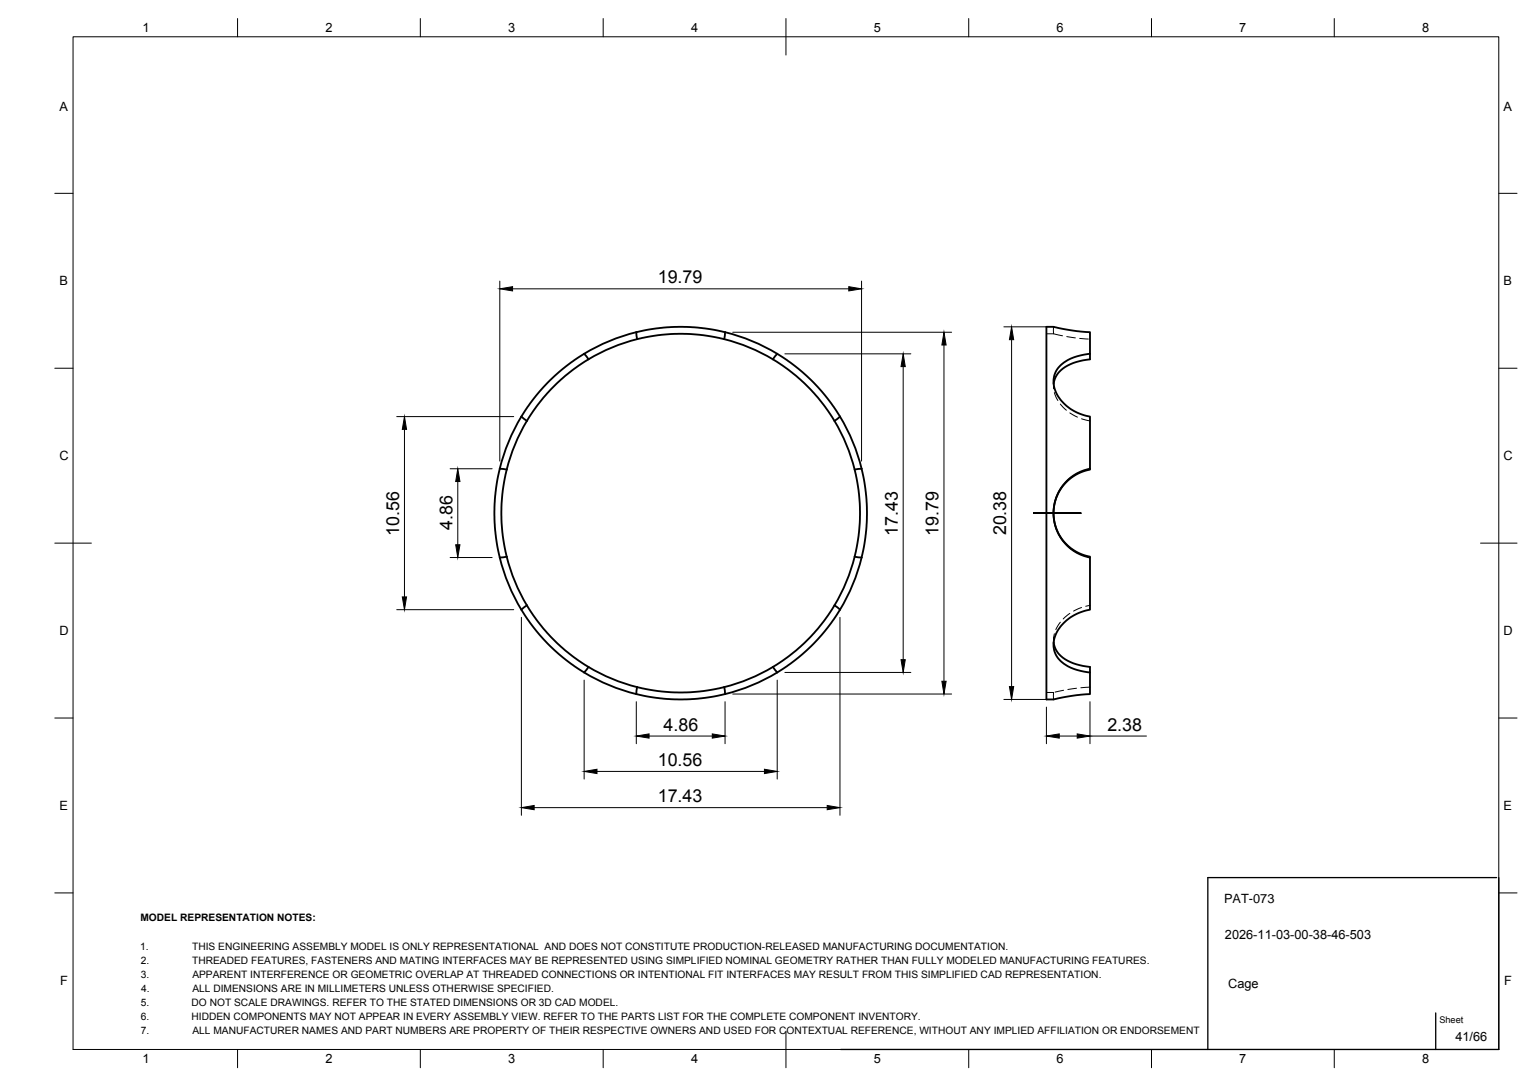
ISO-10303-21;
HEADER;
/* Generated by software containing ST-Developer
 * from STEP Tools, Inc. (www.steptools.com) 
 */

FILE_DESCRIPTION(
/* description */ ('Manual piston pump'),
/* implementation_level */ '2;1');

FILE_NAME(
/* name */ 'Cage.step',
/* time_stamp */ '2026-11-02T16:54:23-08:00',
/* author */ (''),
/* organization */ (''),
/* preprocessor_version */ 'ST-DEVELOPER v20.2',
/* originating_system */ 'Autodesk Translation Framework v15.17.0.0',
/* authorisation */ '');

FILE_SCHEMA (('AUTOMOTIVE_DESIGN { 1 0 10303 214 3 1 1 }'));
ENDSEC;

DATA;
#10=MECHANICAL_DESIGN_GEOMETRIC_PRESENTATION_REPRESENTATION('',(#721),#19043);
#500=SPHERICAL_SURFACE('',#10763,0.247676);
#501=SPHERICAL_SURFACE('',#10779,0.247676);
#502=SPHERICAL_SURFACE('',#10784,0.247676);
#503=SPHERICAL_SURFACE('',#10789,0.247676);
#504=SPHERICAL_SURFACE('',#10794,0.247676);
#505=SPHERICAL_SURFACE('',#10799,0.247676);
#506=SPHERICAL_SURFACE('',#10804,0.247676);
#507=SPHERICAL_SURFACE('',#10812,0.247676);
#588=SHAPE_REPRESENTATION_RELATIONSHIP('SRR','None',#19335,#651);
#651=ADVANCED_BREP_SHAPE_REPRESENTATION('',(#791),#19002);
#721=STYLED_ITEM('',(#19661),#791);
#791=MANIFOLD_SOLID_BREP('Continuous crown cage',#9507);
#950=FACE_BOUND('',#2270,.T.);
#1051=B_SPLINE_CURVE_WITH_KNOTS('',3,(#15858,#15859,#15860,#15861,#15862,
#15863,#15864,#15865,#15866,#15867,#15868,#15869,#15870,#15871,#15872,#15873,
#15874,#15875,#15876,#15877,#15878,#15879),.UNSPECIFIED.,.F.,.F.,(4,2,2,
2,2,2,2,2,2,2,4),(0.0473477652366656,0.126350602536658,0.189525903804987,
0.252701205073317,0.313298422430275,0.373895639787233,0.434492857144191,
0.495090074501149,0.558265375769478,0.621440677037807,0.7004435143378),
 .UNSPECIFIED.);
#1052=B_SPLINE_CURVE_WITH_KNOTS('',3,(#15883,#15884,#15885,#15886,#15887,
#15888,#15889,#15890,#15891,#15892,#15893,#15894,#15895,#15896,#15897,#15898,
#15899,#15900,#15901,#15902,#15903,#15904),.UNSPECIFIED.,.F.,.F.,(4,2,2,
2,2,2,2,2,2,2,4),(0.0464897534940957,0.0852567806515119,0.170513561303024,
0.246687263103517,0.308657850341199,0.370628437578881,0.432599024816563,
0.494569612054245,0.570743313854739,0.656000094506251,0.694767121663666),
 .UNSPECIFIED.);
#1053=B_SPLINE_CURVE_WITH_KNOTS('',3,(#15910,#15911,#15912,#15913,#15914,
#15915,#15916,#15917,#15918,#15919,#15920,#15921,#15922,#15923,#15924,#15925,
#15926,#15927,#15928,#15929,#15930,#15931),.UNSPECIFIED.,.F.,.F.,(4,2,2,
2,2,2,2,2,2,2,4),(0.0464897534940957,0.0852567806515118,0.170513561303024,
0.246687263103517,0.308657850341199,0.370628437578881,0.432599024816563,
0.494569612054245,0.570743313854738,0.65600009450625,0.694767121663666),
 .UNSPECIFIED.);
#1054=B_SPLINE_CURVE_WITH_KNOTS('',3,(#15935,#15936,#15937,#15938,#15939,
#15940,#15941,#15942,#15943,#15944,#15945,#15946,#15947,#15948,#15949,#15950,
#15951,#15952,#15953,#15954,#15955,#15956),.UNSPECIFIED.,.F.,.F.,(4,2,2,
2,2,2,2,2,2,2,4),(0.0464897534940957,0.0852567806515119,0.170513561303024,
0.246687263103517,0.308657850341199,0.370628437578881,0.432599024816563,
0.494569612054245,0.570743313854739,0.656000094506251,0.694767121663666),
 .UNSPECIFIED.);
#1055=B_SPLINE_CURVE_WITH_KNOTS('',3,(#15960,#15961,#15962,#15963,#15964,
#15965,#15966,#15967,#15968,#15969,#15970,#15971),.UNSPECIFIED.,.F.,.F.,
(4,2,2,2,2,4),(0.0464897534940957,0.0852567806515119,0.170513561303024,
0.246687263103517,0.308657850341199,0.370628437578881),.UNSPECIFIED.);
#1056=B_SPLINE_CURVE_WITH_KNOTS('',3,(#15976,#15977,#15978,#15979,#15980,
#15981,#15982,#15983,#15984,#15985,#15986,#15987),.UNSPECIFIED.,.F.,.F.,
(4,2,2,2,2,4),(0.370628437578881,0.432599024816563,0.494569612054245,0.570743313854738,
0.65600009450625,0.694767121663666),.UNSPECIFIED.);
#1057=B_SPLINE_CURVE_WITH_KNOTS('',3,(#15991,#15992,#15993,#15994,#15995,
#15996,#15997,#15998,#15999,#16000,#16001,#16002,#16003,#16004,#16005,#16006,
#16007,#16008,#16009,#16010,#16011,#16012),.UNSPECIFIED.,.F.,.F.,(4,2,2,
2,2,2,2,2,2,2,4),(0.0464897534940957,0.0852567806515121,0.170513561303024,
0.246687263103518,0.308657850341199,0.370628437578881,0.432599024816563,
0.494569612054245,0.570743313854738,0.65600009450625,0.694767121663666),
 .UNSPECIFIED.);
#1058=B_SPLINE_CURVE_WITH_KNOTS('',3,(#16016,#16017,#16018,#16019,#16020,
#16021,#16022,#16023,#16024,#16025,#16026,#16027,#16028,#16029,#16030,#16031,
#16032,#16033,#16034,#16035,#16036,#16037),.UNSPECIFIED.,.F.,.F.,(4,2,2,
2,2,2,2,2,2,2,4),(0.0464897534940957,0.0852567806515119,0.170513561303024,
0.246687263103517,0.308657850341199,0.370628437578881,0.432599024816563,
0.494569612054245,0.570743313854738,0.65600009450625,0.694767121663667),
 .UNSPECIFIED.);
#1059=B_SPLINE_CURVE_WITH_KNOTS('',3,(#16041,#16042,#16043,#16044,#16045,
#16046,#16047,#16048,#16049,#16050,#16051,#16052,#16053,#16054,#16055,#16056,
#16057,#16058,#16059,#16060,#16061,#16062),.UNSPECIFIED.,.F.,.F.,(4,2,2,
2,2,2,2,2,2,2,4),(0.0464897534940957,0.0852567806515119,0.170513561303024,
0.246687263103517,0.308657850341199,0.370628437578881,0.432599024816563,
0.494569612054245,0.570743313854738,0.65600009450625,0.694767121663666),
 .UNSPECIFIED.);
#1060=B_SPLINE_CURVE_WITH_KNOTS('',3,(#16066,#16067,#16068,#16069,#16070,
#16071,#16072,#16073,#16074,#16075,#16076,#16077,#16078,#16079,#16080,#16081,
#16082,#16083,#16084,#16085,#16086,#16087),.UNSPECIFIED.,.F.,.F.,(4,2,2,
2,2,2,2,2,2,2,4),(0.0464897534940957,0.0852567806515119,0.170513561303024,
0.246687263103517,0.308657850341199,0.370628437578881,0.432599024816563,
0.494569612054245,0.570743313854739,0.656000094506251,0.694767121663667),
 .UNSPECIFIED.);
#1061=B_SPLINE_CURVE_WITH_KNOTS('',3,(#16095,#16096,#16097,#16098,#16099,
#16100,#16101,#16102,#16103,#16104,#16105,#16106,#16107,#16108,#16109,#16110,
#16111,#16112,#16113,#16114,#16115,#16116),.UNSPECIFIED.,.F.,.F.,(4,2,2,
2,2,2,2,2,2,2,4),(0.0473477652366656,0.126350602536658,0.189525903804987,
0.252701205073316,0.313298422430274,0.373895639787232,0.434492857144191,
0.495090074501149,0.558265375769478,0.621440677037807,0.7004435143378),
 .UNSPECIFIED.);
#1062=B_SPLINE_CURVE_WITH_KNOTS('',3,(#16124,#16125,#16126,#16127,#16128,
#16129,#16130,#16131,#16132,#16133,#16134,#16135,#16136,#16137,#16138,#16139,
#16140,#16141,#16142,#16143,#16144,#16145),.UNSPECIFIED.,.F.,.F.,(4,2,2,
2,2,2,2,2,2,2,4),(0.0473477652366656,0.126350602536658,0.189525903804987,
0.252701205073317,0.313298422430275,0.373895639787233,0.434492857144191,
0.495090074501149,0.558265375769478,0.621440677037807,0.7004435143378),
 .UNSPECIFIED.);
#1063=B_SPLINE_CURVE_WITH_KNOTS('',3,(#16154,#16155,#16156,#16157,#16158,
#16159,#16160,#16161,#16162,#16163,#16164,#16165),.UNSPECIFIED.,.F.,.F.,
(4,2,2,2,2,4),(0.0473477652366656,0.126350602536658,0.189525903804987,0.252701205073316,
0.313298422430275,0.373895639787233),.UNSPECIFIED.);
#1064=B_SPLINE_CURVE_WITH_KNOTS('',3,(#16167,#16168,#16169,#16170,#16171,
#16172,#16173,#16174,#16175,#16176,#16177,#16178),.UNSPECIFIED.,.F.,.F.,
(4,2,2,2,2,4),(0.373895639787233,0.434492857144191,0.495090074501149,0.558265375769478,
0.621440677037807,0.7004435143378),.UNSPECIFIED.);
#1065=B_SPLINE_CURVE_WITH_KNOTS('',3,(#16185,#16186,#16187,#16188,#16189,
#16190,#16191,#16192,#16193,#16194,#16195,#16196,#16197,#16198,#16199,#16200,
#16201,#16202,#16203,#16204,#16205,#16206),.UNSPECIFIED.,.F.,.F.,(4,2,2,
2,2,2,2,2,2,2,4),(0.0473477652366656,0.126350602536658,0.189525903804987,
0.252701205073316,0.313298422430275,0.373895639787233,0.434492857144191,
0.495090074501149,0.558265375769478,0.621440677037807,0.7004435143378),
 .UNSPECIFIED.);
#1066=B_SPLINE_CURVE_WITH_KNOTS('',3,(#16214,#16215,#16216,#16217,#16218,
#16219,#16220,#16221,#16222,#16223,#16224,#16225,#16226,#16227,#16228,#16229,
#16230,#16231,#16232,#16233,#16234,#16235),.UNSPECIFIED.,.F.,.F.,(4,2,2,
2,2,2,2,2,2,2,4),(0.0473477652366656,0.126350602536658,0.189525903804987,
0.252701205073317,0.313298422430275,0.373895639787233,0.434492857144191,
0.495090074501149,0.558265375769478,0.621440677037807,0.7004435143378),
 .UNSPECIFIED.);
#1067=B_SPLINE_CURVE_WITH_KNOTS('',3,(#16243,#16244,#16245,#16246,#16247,
#16248,#16249,#16250,#16251,#16252,#16253,#16254,#16255,#16256,#16257,#16258,
#16259,#16260,#16261,#16262,#16263,#16264),.UNSPECIFIED.,.F.,.F.,(4,2,2,
2,2,2,2,2,2,2,4),(0.0473477652366656,0.126350602536658,0.189525903804987,
0.252701205073316,0.313298422430275,0.373895639787233,0.434492857144191,
0.495090074501149,0.558265375769478,0.621440677037807,0.7004435143378),
 .UNSPECIFIED.);
#1068=B_SPLINE_CURVE_WITH_KNOTS('',3,(#16273,#16274,#16275,#16276,#16277,
#16278,#16279,#16280,#16281,#16282,#16283,#16284,#16285,#16286,#16287,#16288,
#16289,#16290,#16291,#16292,#16293,#16294),.UNSPECIFIED.,.F.,.F.,(4,2,2,
2,2,2,2,2,2,2,4),(0.0473477652366656,0.126350602536658,0.189525903804987,
0.252701205073317,0.313298422430275,0.373895639787233,0.434492857144191,
0.495090074501149,0.558265375769478,0.621440677037807,0.7004435143378),
 .UNSPECIFIED.);
#1189=CYLINDRICAL_SURFACE('',#10766,1.019052);
#1190=CYLINDRICAL_SURFACE('',#10806,0.980948);
#1554=FACE_OUTER_BOUND('',#2252,.T.);
#1555=FACE_OUTER_BOUND('',#2253,.T.);
#1556=FACE_OUTER_BOUND('',#2254,.T.);
#1557=FACE_OUTER_BOUND('',#2255,.T.);
#1558=FACE_OUTER_BOUND('',#2256,.T.);
#1559=FACE_OUTER_BOUND('',#2257,.T.);
#1560=FACE_OUTER_BOUND('',#2258,.T.);
#1561=FACE_OUTER_BOUND('',#2259,.T.);
#1562=FACE_OUTER_BOUND('',#2260,.T.);
#1563=FACE_OUTER_BOUND('',#2261,.T.);
#1564=FACE_OUTER_BOUND('',#2262,.T.);
#1565=FACE_OUTER_BOUND('',#2263,.T.);
#1566=FACE_OUTER_BOUND('',#2264,.T.);
#1567=FACE_OUTER_BOUND('',#2265,.T.);
#1568=FACE_OUTER_BOUND('',#2266,.T.);
#1569=FACE_OUTER_BOUND('',#2267,.T.);
#1570=FACE_OUTER_BOUND('',#2268,.T.);
#1571=FACE_OUTER_BOUND('',#2269,.T.);
#1572=FACE_OUTER_BOUND('',#2271,.T.);
#2252=EDGE_LOOP('',(#7329,#7330,#7331,#7332));
#2253=EDGE_LOOP('',(#7333,#7334,#7335,#7336,#7337,#7338,#7339,#7340,#7341,
#7342,#7343,#7344,#7345,#7346,#7347,#7348,#7349,#7350,#7351,#7352));
#2254=EDGE_LOOP('',(#7353,#7354,#7355,#7356));
#2255=EDGE_LOOP('',(#7357,#7358,#7359,#7360));
#2256=EDGE_LOOP('',(#7361,#7362,#7363,#7364));
#2257=EDGE_LOOP('',(#7365,#7366,#7367,#7368));
#2258=EDGE_LOOP('',(#7369,#7370,#7371,#7372));
#2259=EDGE_LOOP('',(#7373,#7374,#7375,#7376,#7377,#7378));
#2260=EDGE_LOOP('',(#7379,#7380,#7381,#7382));
#2261=EDGE_LOOP('',(#7383,#7384,#7385,#7386));
#2262=EDGE_LOOP('',(#7387,#7388,#7389,#7390));
#2263=EDGE_LOOP('',(#7391,#7392,#7393,#7394));
#2264=EDGE_LOOP('',(#7395,#7396,#7397,#7398));
#2265=EDGE_LOOP('',(#7399,#7400,#7401,#7402));
#2266=EDGE_LOOP('',(#7403,#7404,#7405,#7406,#7407,#7408,#7409,#7410,#7411,
#7412,#7413,#7414,#7415,#7416,#7417,#7418,#7419,#7420,#7421,#7422));
#2267=EDGE_LOOP('',(#7423,#7424,#7425,#7426));
#2268=EDGE_LOOP('',(#7427,#7428,#7429,#7430));
#2269=EDGE_LOOP('',(#7431));
#2270=EDGE_LOOP('',(#7432));
#2271=EDGE_LOOP('',(#7433,#7434,#7435,#7436));
#2891=CIRCLE('',#10764,0.243053047864041);
#2892=CIRCLE('',#10765,0.243053047864041);
#2893=CIRCLE('',#10767,1.019052);
#2894=CIRCLE('',#10768,1.019052);
#2895=CIRCLE('',#10769,1.019052);
#2896=CIRCLE('',#10770,1.019052);
#2897=CIRCLE('',#10771,1.019052);
#2898=CIRCLE('',#10772,1.019052);
#2899=CIRCLE('',#10773,1.019052);
#2900=CIRCLE('',#10774,1.019052);
#2901=CIRCLE('',#10775,1.019052);
#2902=CIRCLE('',#10777,0.980948);
#2903=CIRCLE('',#10778,0.243053047864041);
#2904=CIRCLE('',#10780,0.243053047864041);
#2905=CIRCLE('',#10782,0.980948);
#2906=CIRCLE('',#10783,0.243053047864041);
#2907=CIRCLE('',#10785,0.243053047864041);
#2908=CIRCLE('',#10787,0.980948);
#2909=CIRCLE('',#10788,0.243053047864041);
#2910=CIRCLE('',#10790,0.243053047864041);
#2911=CIRCLE('',#10792,0.980948);
#2912=CIRCLE('',#10793,0.243053047864041);
#2913=CIRCLE('',#10795,0.243053047864041);
#2914=CIRCLE('',#10797,0.980948);
#2915=CIRCLE('',#10798,0.243053047864041);
#2916=CIRCLE('',#10800,0.243053047864041);
#2917=CIRCLE('',#10802,0.980948);
#2918=CIRCLE('',#10803,0.243053047864041);
#2919=CIRCLE('',#10805,0.243053047864041);
#2920=CIRCLE('',#10807,0.980948);
#2921=CIRCLE('',#10808,0.980948);
#2922=CIRCLE('',#10809,0.980948);
#2923=CIRCLE('',#10811,0.243053047864041);
#2924=CIRCLE('',#10813,0.243053047864041);
#3432=LINE('',#15973,#4036);
#3433=LINE('',#16269,#4037);
#4036=VECTOR('',#12834,1.019052);
#4037=VECTOR('',#12911,0.980948);
#4712=VERTEX_POINT('',#15856);
#4713=VERTEX_POINT('',#15857);
#4714=VERTEX_POINT('',#15880);
#4715=VERTEX_POINT('',#15882);
#4716=VERTEX_POINT('',#15907);
#4717=VERTEX_POINT('',#15909);
#4718=VERTEX_POINT('',#15932);
#4719=VERTEX_POINT('',#15934);
#4720=VERTEX_POINT('',#15957);
#4721=VERTEX_POINT('',#15959);
#4722=VERTEX_POINT('',#15972);
#4723=VERTEX_POINT('',#15975);
#4724=VERTEX_POINT('',#15988);
#4725=VERTEX_POINT('',#15990);
#4726=VERTEX_POINT('',#16013);
#4727=VERTEX_POINT('',#16015);
#4728=VERTEX_POINT('',#16038);
#4729=VERTEX_POINT('',#16040);
#4730=VERTEX_POINT('',#16063);
#4731=VERTEX_POINT('',#16065);
#4732=VERTEX_POINT('',#16090);
#4733=VERTEX_POINT('',#16094);
#4734=VERTEX_POINT('',#16119);
#4735=VERTEX_POINT('',#16123);
#4736=VERTEX_POINT('',#16148);
#4737=VERTEX_POINT('',#16152);
#4738=VERTEX_POINT('',#16153);
#4739=VERTEX_POINT('',#16180);
#4740=VERTEX_POINT('',#16184);
#4741=VERTEX_POINT('',#16209);
#4742=VERTEX_POINT('',#16213);
#4743=VERTEX_POINT('',#16238);
#4744=VERTEX_POINT('',#16242);
#4745=VERTEX_POINT('',#16267);
#4746=VERTEX_POINT('',#16270);
#4747=VERTEX_POINT('',#16272);
#5651=EDGE_CURVE('',#4712,#4713,#1051,.T.);
#5652=EDGE_CURVE('',#4714,#4712,#2891,.T.);
#5653=EDGE_CURVE('',#4715,#4714,#1052,.T.);
#5654=EDGE_CURVE('',#4713,#4715,#2892,.T.);
#5655=EDGE_CURVE('',#4716,#4714,#2893,.T.);
#5656=EDGE_CURVE('',#4716,#4717,#1053,.T.);
#5657=EDGE_CURVE('',#4718,#4717,#2894,.T.);
#5658=EDGE_CURVE('',#4718,#4719,#1054,.T.);
#5659=EDGE_CURVE('',#4720,#4719,#2895,.T.);
#5660=EDGE_CURVE('',#4720,#4721,#1055,.T.);
#5661=EDGE_CURVE('',#4721,#4722,#3432,.T.);
#5662=EDGE_CURVE('',#4722,#4722,#2896,.T.);
#5663=EDGE_CURVE('',#4721,#4723,#1056,.T.);
#5664=EDGE_CURVE('',#4724,#4723,#2897,.T.);
#5665=EDGE_CURVE('',#4724,#4725,#1057,.T.);
#5666=EDGE_CURVE('',#4726,#4725,#2898,.T.);
#5667=EDGE_CURVE('',#4726,#4727,#1058,.T.);
#5668=EDGE_CURVE('',#4728,#4727,#2899,.T.);
#5669=EDGE_CURVE('',#4728,#4729,#1059,.T.);
#5670=EDGE_CURVE('',#4730,#4729,#2900,.T.);
#5671=EDGE_CURVE('',#4730,#4731,#1060,.T.);
#5672=EDGE_CURVE('',#4715,#4731,#2901,.T.);
#5673=EDGE_CURVE('',#4712,#4732,#2902,.T.);
#5674=EDGE_CURVE('',#4732,#4716,#2903,.T.);
#5675=EDGE_CURVE('',#4733,#4732,#1061,.T.);
#5676=EDGE_CURVE('',#4717,#4733,#2904,.T.);
#5677=EDGE_CURVE('',#4733,#4734,#2905,.T.);
#5678=EDGE_CURVE('',#4734,#4718,#2906,.T.);
#5679=EDGE_CURVE('',#4735,#4734,#1062,.T.);
#5680=EDGE_CURVE('',#4719,#4735,#2907,.T.);
#5681=EDGE_CURVE('',#4735,#4736,#2908,.T.);
#5682=EDGE_CURVE('',#4736,#4720,#2909,.T.);
#5683=EDGE_CURVE('',#4737,#4738,#1063,.T.);
#5684=EDGE_CURVE('',#4723,#4737,#2910,.T.);
#5685=EDGE_CURVE('',#4738,#4736,#1064,.T.);
#5686=EDGE_CURVE('',#4737,#4739,#2911,.T.);
#5687=EDGE_CURVE('',#4739,#4724,#2912,.T.);
#5688=EDGE_CURVE('',#4740,#4739,#1065,.T.);
#5689=EDGE_CURVE('',#4725,#4740,#2913,.T.);
#5690=EDGE_CURVE('',#4740,#4741,#2914,.T.);
#5691=EDGE_CURVE('',#4741,#4726,#2915,.T.);
#5692=EDGE_CURVE('',#4742,#4741,#1066,.T.);
#5693=EDGE_CURVE('',#4727,#4742,#2916,.T.);
#5694=EDGE_CURVE('',#4742,#4743,#2917,.T.);
#5695=EDGE_CURVE('',#4743,#4728,#2918,.T.);
#5696=EDGE_CURVE('',#4744,#4743,#1067,.T.);
#5697=EDGE_CURVE('',#4729,#4744,#2919,.T.);
#5698=EDGE_CURVE('',#4745,#4745,#2920,.T.);
#5699=EDGE_CURVE('',#4745,#4738,#3433,.T.);
#5700=EDGE_CURVE('',#4746,#4713,#2921,.T.);
#5701=EDGE_CURVE('',#4746,#4747,#1068,.T.);
#5702=EDGE_CURVE('',#4744,#4747,#2922,.T.);
#5703=EDGE_CURVE('',#4731,#4746,#2923,.T.);
#5704=EDGE_CURVE('',#4747,#4730,#2924,.T.);
#7329=ORIENTED_EDGE('',*,*,#5651,.F.);
#7330=ORIENTED_EDGE('',*,*,#5652,.F.);
#7331=ORIENTED_EDGE('',*,*,#5653,.F.);
#7332=ORIENTED_EDGE('',*,*,#5654,.F.);
#7333=ORIENTED_EDGE('',*,*,#5653,.T.);
#7334=ORIENTED_EDGE('',*,*,#5655,.F.);
#7335=ORIENTED_EDGE('',*,*,#5656,.T.);
#7336=ORIENTED_EDGE('',*,*,#5657,.F.);
#7337=ORIENTED_EDGE('',*,*,#5658,.T.);
#7338=ORIENTED_EDGE('',*,*,#5659,.F.);
#7339=ORIENTED_EDGE('',*,*,#5660,.T.);
#7340=ORIENTED_EDGE('',*,*,#5661,.T.);
#7341=ORIENTED_EDGE('',*,*,#5662,.F.);
#7342=ORIENTED_EDGE('',*,*,#5661,.F.);
#7343=ORIENTED_EDGE('',*,*,#5663,.T.);
#7344=ORIENTED_EDGE('',*,*,#5664,.F.);
#7345=ORIENTED_EDGE('',*,*,#5665,.T.);
#7346=ORIENTED_EDGE('',*,*,#5666,.F.);
#7347=ORIENTED_EDGE('',*,*,#5667,.T.);
#7348=ORIENTED_EDGE('',*,*,#5668,.F.);
#7349=ORIENTED_EDGE('',*,*,#5669,.T.);
#7350=ORIENTED_EDGE('',*,*,#5670,.F.);
#7351=ORIENTED_EDGE('',*,*,#5671,.T.);
#7352=ORIENTED_EDGE('',*,*,#5672,.F.);
#7353=ORIENTED_EDGE('',*,*,#5652,.T.);
#7354=ORIENTED_EDGE('',*,*,#5673,.T.);
#7355=ORIENTED_EDGE('',*,*,#5674,.T.);
#7356=ORIENTED_EDGE('',*,*,#5655,.T.);
#7357=ORIENTED_EDGE('',*,*,#5675,.F.);
#7358=ORIENTED_EDGE('',*,*,#5676,.F.);
#7359=ORIENTED_EDGE('',*,*,#5656,.F.);
#7360=ORIENTED_EDGE('',*,*,#5674,.F.);
#7361=ORIENTED_EDGE('',*,*,#5676,.T.);
#7362=ORIENTED_EDGE('',*,*,#5677,.T.);
#7363=ORIENTED_EDGE('',*,*,#5678,.T.);
#7364=ORIENTED_EDGE('',*,*,#5657,.T.);
#7365=ORIENTED_EDGE('',*,*,#5679,.F.);
#7366=ORIENTED_EDGE('',*,*,#5680,.F.);
#7367=ORIENTED_EDGE('',*,*,#5658,.F.);
#7368=ORIENTED_EDGE('',*,*,#5678,.F.);
#7369=ORIENTED_EDGE('',*,*,#5680,.T.);
#7370=ORIENTED_EDGE('',*,*,#5681,.T.);
#7371=ORIENTED_EDGE('',*,*,#5682,.T.);
#7372=ORIENTED_EDGE('',*,*,#5659,.T.);
#7373=ORIENTED_EDGE('',*,*,#5683,.F.);
#7374=ORIENTED_EDGE('',*,*,#5684,.F.);
#7375=ORIENTED_EDGE('',*,*,#5663,.F.);
#7376=ORIENTED_EDGE('',*,*,#5660,.F.);
#7377=ORIENTED_EDGE('',*,*,#5682,.F.);
#7378=ORIENTED_EDGE('',*,*,#5685,.F.);
#7379=ORIENTED_EDGE('',*,*,#5684,.T.);
#7380=ORIENTED_EDGE('',*,*,#5686,.T.);
#7381=ORIENTED_EDGE('',*,*,#5687,.T.);
#7382=ORIENTED_EDGE('',*,*,#5664,.T.);
#7383=ORIENTED_EDGE('',*,*,#5688,.F.);
#7384=ORIENTED_EDGE('',*,*,#5689,.F.);
#7385=ORIENTED_EDGE('',*,*,#5665,.F.);
#7386=ORIENTED_EDGE('',*,*,#5687,.F.);
#7387=ORIENTED_EDGE('',*,*,#5689,.T.);
#7388=ORIENTED_EDGE('',*,*,#5690,.T.);
#7389=ORIENTED_EDGE('',*,*,#5691,.T.);
#7390=ORIENTED_EDGE('',*,*,#5666,.T.);
#7391=ORIENTED_EDGE('',*,*,#5692,.F.);
#7392=ORIENTED_EDGE('',*,*,#5693,.F.);
#7393=ORIENTED_EDGE('',*,*,#5667,.F.);
#7394=ORIENTED_EDGE('',*,*,#5691,.F.);
#7395=ORIENTED_EDGE('',*,*,#5693,.T.);
#7396=ORIENTED_EDGE('',*,*,#5694,.T.);
#7397=ORIENTED_EDGE('',*,*,#5695,.T.);
#7398=ORIENTED_EDGE('',*,*,#5668,.T.);
#7399=ORIENTED_EDGE('',*,*,#5669,.F.);
#7400=ORIENTED_EDGE('',*,*,#5695,.F.);
#7401=ORIENTED_EDGE('',*,*,#5696,.F.);
#7402=ORIENTED_EDGE('',*,*,#5697,.F.);
#7403=ORIENTED_EDGE('',*,*,#5698,.F.);
#7404=ORIENTED_EDGE('',*,*,#5699,.T.);
#7405=ORIENTED_EDGE('',*,*,#5685,.T.);
#7406=ORIENTED_EDGE('',*,*,#5681,.F.);
#7407=ORIENTED_EDGE('',*,*,#5679,.T.);
#7408=ORIENTED_EDGE('',*,*,#5677,.F.);
#7409=ORIENTED_EDGE('',*,*,#5675,.T.);
#7410=ORIENTED_EDGE('',*,*,#5673,.F.);
#7411=ORIENTED_EDGE('',*,*,#5651,.T.);
#7412=ORIENTED_EDGE('',*,*,#5700,.F.);
#7413=ORIENTED_EDGE('',*,*,#5701,.T.);
#7414=ORIENTED_EDGE('',*,*,#5702,.F.);
#7415=ORIENTED_EDGE('',*,*,#5696,.T.);
#7416=ORIENTED_EDGE('',*,*,#5694,.F.);
#7417=ORIENTED_EDGE('',*,*,#5692,.T.);
#7418=ORIENTED_EDGE('',*,*,#5690,.F.);
#7419=ORIENTED_EDGE('',*,*,#5688,.T.);
#7420=ORIENTED_EDGE('',*,*,#5686,.F.);
#7421=ORIENTED_EDGE('',*,*,#5683,.T.);
#7422=ORIENTED_EDGE('',*,*,#5699,.F.);
#7423=ORIENTED_EDGE('',*,*,#5654,.T.);
#7424=ORIENTED_EDGE('',*,*,#5672,.T.);
#7425=ORIENTED_EDGE('',*,*,#5703,.T.);
#7426=ORIENTED_EDGE('',*,*,#5700,.T.);
#7427=ORIENTED_EDGE('',*,*,#5671,.F.);
#7428=ORIENTED_EDGE('',*,*,#5704,.F.);
#7429=ORIENTED_EDGE('',*,*,#5701,.F.);
#7430=ORIENTED_EDGE('',*,*,#5703,.F.);
#7431=ORIENTED_EDGE('',*,*,#5662,.T.);
#7432=ORIENTED_EDGE('',*,*,#5698,.T.);
#7433=ORIENTED_EDGE('',*,*,#5697,.T.);
#7434=ORIENTED_EDGE('',*,*,#5702,.T.);
#7435=ORIENTED_EDGE('',*,*,#5704,.T.);
#7436=ORIENTED_EDGE('',*,*,#5670,.T.);
#8712=PLANE('',#10776);
#8713=PLANE('',#10781);
#8714=PLANE('',#10786);
#8715=PLANE('',#10791);
#8716=PLANE('',#10796);
#8717=PLANE('',#10801);
#8718=PLANE('',#10810);
#8719=PLANE('',#10814);
#8720=PLANE('',#10815);
#9159=ADVANCED_FACE('',(#1554),#500,.F.);
#9160=ADVANCED_FACE('',(#1555),#1189,.T.);
#9161=ADVANCED_FACE('',(#1556),#8712,.T.);
#9162=ADVANCED_FACE('',(#1557),#501,.F.);
#9163=ADVANCED_FACE('',(#1558),#8713,.T.);
#9164=ADVANCED_FACE('',(#1559),#502,.F.);
#9165=ADVANCED_FACE('',(#1560),#8714,.T.);
#9166=ADVANCED_FACE('',(#1561),#503,.F.);
#9167=ADVANCED_FACE('',(#1562),#8715,.T.);
#9168=ADVANCED_FACE('',(#1563),#504,.F.);
#9169=ADVANCED_FACE('',(#1564),#8716,.T.);
#9170=ADVANCED_FACE('',(#1565),#505,.F.);
#9171=ADVANCED_FACE('',(#1566),#8717,.T.);
#9172=ADVANCED_FACE('',(#1567),#506,.F.);
#9173=ADVANCED_FACE('',(#1568),#1190,.F.);
#9174=ADVANCED_FACE('',(#1569),#8718,.T.);
#9175=ADVANCED_FACE('',(#1570),#507,.F.);
#9176=ADVANCED_FACE('',(#1571,#950),#8719,.T.);
#9177=ADVANCED_FACE('',(#1572),#8720,.T.);
#9507=CLOSED_SHELL('',(#9159,#9160,#9161,#9162,#9163,#9164,#9165,#9166,
#9167,#9168,#9169,#9170,#9171,#9172,#9173,#9174,#9175,#9176,#9177));
#10762=AXIS2_PLACEMENT_3D('',#15854,#12818,#12819);
#10763=AXIS2_PLACEMENT_3D('',#15855,#12820,#12821);
#10764=AXIS2_PLACEMENT_3D('',#15881,#12822,#12823);
#10765=AXIS2_PLACEMENT_3D('',#15905,#12824,#12825);
#10766=AXIS2_PLACEMENT_3D('',#15906,#12826,#12827);
#10767=AXIS2_PLACEMENT_3D('',#15908,#12828,#12829);
#10768=AXIS2_PLACEMENT_3D('',#15933,#12830,#12831);
#10769=AXIS2_PLACEMENT_3D('',#15958,#12832,#12833);
#10770=AXIS2_PLACEMENT_3D('',#15974,#12835,#12836);
#10771=AXIS2_PLACEMENT_3D('',#15989,#12837,#12838);
#10772=AXIS2_PLACEMENT_3D('',#16014,#12839,#12840);
#10773=AXIS2_PLACEMENT_3D('',#16039,#12841,#12842);
#10774=AXIS2_PLACEMENT_3D('',#16064,#12843,#12844);
#10775=AXIS2_PLACEMENT_3D('',#16088,#12845,#12846);
#10776=AXIS2_PLACEMENT_3D('',#16089,#12847,#12848);
#10777=AXIS2_PLACEMENT_3D('',#16091,#12849,#12850);
#10778=AXIS2_PLACEMENT_3D('',#16092,#12851,#12852);
#10779=AXIS2_PLACEMENT_3D('',#16093,#12853,#12854);
#10780=AXIS2_PLACEMENT_3D('',#16117,#12855,#12856);
#10781=AXIS2_PLACEMENT_3D('',#16118,#12857,#12858);
#10782=AXIS2_PLACEMENT_3D('',#16120,#12859,#12860);
#10783=AXIS2_PLACEMENT_3D('',#16121,#12861,#12862);
#10784=AXIS2_PLACEMENT_3D('',#16122,#12863,#12864);
#10785=AXIS2_PLACEMENT_3D('',#16146,#12865,#12866);
#10786=AXIS2_PLACEMENT_3D('',#16147,#12867,#12868);
#10787=AXIS2_PLACEMENT_3D('',#16149,#12869,#12870);
#10788=AXIS2_PLACEMENT_3D('',#16150,#12871,#12872);
#10789=AXIS2_PLACEMENT_3D('',#16151,#12873,#12874);
#10790=AXIS2_PLACEMENT_3D('',#16166,#12875,#12876);
#10791=AXIS2_PLACEMENT_3D('',#16179,#12877,#12878);
#10792=AXIS2_PLACEMENT_3D('',#16181,#12879,#12880);
#10793=AXIS2_PLACEMENT_3D('',#16182,#12881,#12882);
#10794=AXIS2_PLACEMENT_3D('',#16183,#12883,#12884);
#10795=AXIS2_PLACEMENT_3D('',#16207,#12885,#12886);
#10796=AXIS2_PLACEMENT_3D('',#16208,#12887,#12888);
#10797=AXIS2_PLACEMENT_3D('',#16210,#12889,#12890);
#10798=AXIS2_PLACEMENT_3D('',#16211,#12891,#12892);
#10799=AXIS2_PLACEMENT_3D('',#16212,#12893,#12894);
#10800=AXIS2_PLACEMENT_3D('',#16236,#12895,#12896);
#10801=AXIS2_PLACEMENT_3D('',#16237,#12897,#12898);
#10802=AXIS2_PLACEMENT_3D('',#16239,#12899,#12900);
#10803=AXIS2_PLACEMENT_3D('',#16240,#12901,#12902);
#10804=AXIS2_PLACEMENT_3D('',#16241,#12903,#12904);
#10805=AXIS2_PLACEMENT_3D('',#16265,#12905,#12906);
#10806=AXIS2_PLACEMENT_3D('',#16266,#12907,#12908);
#10807=AXIS2_PLACEMENT_3D('',#16268,#12909,#12910);
#10808=AXIS2_PLACEMENT_3D('',#16271,#12912,#12913);
#10809=AXIS2_PLACEMENT_3D('',#16295,#12914,#12915);
#10810=AXIS2_PLACEMENT_3D('',#16296,#12916,#12917);
#10811=AXIS2_PLACEMENT_3D('',#16297,#12918,#12919);
#10812=AXIS2_PLACEMENT_3D('',#16298,#12920,#12921);
#10813=AXIS2_PLACEMENT_3D('',#16299,#12922,#12923);
#10814=AXIS2_PLACEMENT_3D('',#16300,#12924,#12925);
#10815=AXIS2_PLACEMENT_3D('',#16301,#12926,#12927);
#12818=DIRECTION('axis',(0.,0.,1.));
#12819=DIRECTION('refdir',(1.,0.,0.));
#12820=DIRECTION('center_axis',(0.,0.,1.));
#12821=DIRECTION('ref_axis',(1.,0.,0.));
#12822=DIRECTION('center_axis',(0.,-1.,0.));
#12823=DIRECTION('ref_axis',(0.,0.,-1.));
#12824=DIRECTION('center_axis',(0.,-1.,0.));
#12825=DIRECTION('ref_axis',(0.,0.,-1.));
#12826=DIRECTION('center_axis',(0.,1.,0.));
#12827=DIRECTION('ref_axis',(1.,0.,0.));
#12828=DIRECTION('center_axis',(0.,1.,0.));
#12829=DIRECTION('ref_axis',(1.,0.,0.));
#12830=DIRECTION('center_axis',(0.,1.,0.));
#12831=DIRECTION('ref_axis',(1.,0.,0.));
#12832=DIRECTION('center_axis',(0.,1.,0.));
#12833=DIRECTION('ref_axis',(1.,0.,0.));
#12834=DIRECTION('',(0.,-1.,0.));
#12835=DIRECTION('center_axis',(0.,-1.,0.));
#12836=DIRECTION('ref_axis',(1.,0.,0.));
#12837=DIRECTION('center_axis',(0.,1.,0.));
#12838=DIRECTION('ref_axis',(1.,0.,0.));
#12839=DIRECTION('center_axis',(0.,1.,0.));
#12840=DIRECTION('ref_axis',(1.,0.,0.));
#12841=DIRECTION('center_axis',(0.,1.,0.));
#12842=DIRECTION('ref_axis',(1.,0.,0.));
#12843=DIRECTION('center_axis',(0.,1.,0.));
#12844=DIRECTION('ref_axis',(1.,0.,0.));
#12845=DIRECTION('center_axis',(0.,1.,0.));
#12846=DIRECTION('ref_axis',(1.,0.,0.));
#12847=DIRECTION('center_axis',(0.,1.,0.));
#12848=DIRECTION('ref_axis',(1.,0.,0.));
#12849=DIRECTION('center_axis',(0.,-1.,0.));
#12850=DIRECTION('ref_axis',(1.,0.,0.));
#12851=DIRECTION('center_axis',(0.,-1.,0.));
#12852=DIRECTION('ref_axis',(0.,0.,-1.));
#12853=DIRECTION('center_axis',(6.12323399573677E-17,0.,1.));
#12854=DIRECTION('ref_axis',(1.,0.,0.));
#12855=DIRECTION('center_axis',(0.,-1.,0.));
#12856=DIRECTION('ref_axis',(0.,0.,-1.));
#12857=DIRECTION('center_axis',(0.,1.,0.));
#12858=DIRECTION('ref_axis',(1.,0.,0.));
#12859=DIRECTION('center_axis',(0.,-1.,0.));
#12860=DIRECTION('ref_axis',(1.,0.,0.));
#12861=DIRECTION('center_axis',(0.,-1.,0.));
#12862=DIRECTION('ref_axis',(0.,0.,-1.));
#12863=DIRECTION('center_axis',(0.,0.,1.));
#12864=DIRECTION('ref_axis',(1.,0.,0.));
#12865=DIRECTION('center_axis',(0.,-1.,0.));
#12866=DIRECTION('ref_axis',(0.,0.,-1.));
#12867=DIRECTION('center_axis',(0.,1.,0.));
#12868=DIRECTION('ref_axis',(1.,0.,0.));
#12869=DIRECTION('center_axis',(0.,-1.,0.));
#12870=DIRECTION('ref_axis',(1.,0.,0.));
#12871=DIRECTION('center_axis',(0.,-1.,0.));
#12872=DIRECTION('ref_axis',(0.,0.,-1.));
#12873=DIRECTION('center_axis',(0.,0.,1.));
#12874=DIRECTION('ref_axis',(1.,0.,0.));
#12875=DIRECTION('center_axis',(0.,-1.,0.));
#12876=DIRECTION('ref_axis',(0.,0.,-1.));
#12877=DIRECTION('center_axis',(0.,1.,0.));
#12878=DIRECTION('ref_axis',(1.,0.,0.));
#12879=DIRECTION('center_axis',(0.,-1.,0.));
#12880=DIRECTION('ref_axis',(1.,0.,0.));
#12881=DIRECTION('center_axis',(0.,-1.,0.));
#12882=DIRECTION('ref_axis',(0.,0.,-1.));
#12883=DIRECTION('center_axis',(0.,0.,1.));
#12884=DIRECTION('ref_axis',(1.,0.,0.));
#12885=DIRECTION('center_axis',(0.,-1.,0.));
#12886=DIRECTION('ref_axis',(0.,0.,-1.));
#12887=DIRECTION('center_axis',(0.,1.,0.));
#12888=DIRECTION('ref_axis',(1.,0.,0.));
#12889=DIRECTION('center_axis',(0.,-1.,0.));
#12890=DIRECTION('ref_axis',(1.,0.,0.));
#12891=DIRECTION('center_axis',(0.,-1.,0.));
#12892=DIRECTION('ref_axis',(0.,0.,-1.));
#12893=DIRECTION('center_axis',(6.12323399573676E-17,0.,1.));
#12894=DIRECTION('ref_axis',(1.,0.,0.));
#12895=DIRECTION('center_axis',(0.,-1.,0.));
#12896=DIRECTION('ref_axis',(0.,0.,-1.));
#12897=DIRECTION('center_axis',(0.,1.,0.));
#12898=DIRECTION('ref_axis',(1.,0.,0.));
#12899=DIRECTION('center_axis',(0.,-1.,0.));
#12900=DIRECTION('ref_axis',(1.,0.,0.));
#12901=DIRECTION('center_axis',(0.,-1.,0.));
#12902=DIRECTION('ref_axis',(0.,0.,-1.));
#12903=DIRECTION('center_axis',(0.,0.,1.));
#12904=DIRECTION('ref_axis',(1.,0.,0.));
#12905=DIRECTION('center_axis',(0.,-1.,0.));
#12906=DIRECTION('ref_axis',(0.,0.,-1.));
#12907=DIRECTION('center_axis',(0.,1.,0.));
#12908=DIRECTION('ref_axis',(1.,0.,0.));
#12909=DIRECTION('center_axis',(0.,1.,0.));
#12910=DIRECTION('ref_axis',(1.,0.,0.));
#12911=DIRECTION('',(0.,1.,0.));
#12912=DIRECTION('center_axis',(0.,-1.,0.));
#12913=DIRECTION('ref_axis',(1.,0.,0.));
#12914=DIRECTION('center_axis',(0.,-1.,0.));
#12915=DIRECTION('ref_axis',(1.,0.,0.));
#12916=DIRECTION('center_axis',(0.,1.,0.));
#12917=DIRECTION('ref_axis',(1.,0.,0.));
#12918=DIRECTION('center_axis',(0.,-1.,0.));
#12919=DIRECTION('ref_axis',(0.,0.,-1.));
#12920=DIRECTION('center_axis',(0.,0.,1.));
#12921=DIRECTION('ref_axis',(1.,0.,0.));
#12922=DIRECTION('center_axis',(0.,-1.,0.));
#12923=DIRECTION('ref_axis',(0.,0.,-1.));
#12924=DIRECTION('center_axis',(0.,-1.,0.));
#12925=DIRECTION('ref_axis',(-1.,0.,0.));
#12926=DIRECTION('center_axis',(0.,1.,0.));
#12927=DIRECTION('ref_axis',(1.,0.,0.));
#15854=CARTESIAN_POINT('',(0.,0.,0.));
#15855=CARTESIAN_POINT('Origin',(0.707106781186547,0.,0.707106781186548));
#15856=CARTESIAN_POINT('',(0.504455939115715,-0.04763,0.841298510752802));
#15857=CARTESIAN_POINT('',(0.841298510752802,-0.04763,0.504455939115715));
#15858=CARTESIAN_POINT('Ctrl Pts',(0.504455939115715,-0.04763,0.841298510752802));
#15859=CARTESIAN_POINT('Ctrl Pts',(0.508899795931835,-0.0740444353928835,
0.838633903678357));
#15860=CARTESIAN_POINT('Ctrl Pts',(0.517157748491652,-0.0999305678883309,
0.833661031856294));
#15861=CARTESIAN_POINT('Ctrl Pts',(0.537715343527944,-0.142345102874864,
0.820511285096538));
#15862=CARTESIAN_POINT('Ctrl Pts',(0.548874290046456,-0.159766064500479,
0.813159949759));
#15863=CARTESIAN_POINT('Ctrl Pts',(0.573915184558107,-0.190326085855194,
0.795684265985089));
#15864=CARTESIAN_POINT('Ctrl Pts',(0.587792702767295,-0.203463743702801,
0.78555112003688));
#15865=CARTESIAN_POINT('Ctrl Pts',(0.615966552324775,-0.224161999508995,
0.763642258217233));
#15866=CARTESIAN_POINT('Ctrl Pts',(0.631684198665438,-0.232861760990032,
0.750785745543687));
#15867=CARTESIAN_POINT('Ctrl Pts',(0.663382628119203,-0.244251601209411,
0.722929908501543));
#15868=CARTESIAN_POINT('Ctrl Pts',(0.679352081686668,-0.246942143572133,
0.707917883896095));
#15869=CARTESIAN_POINT('Ctrl Pts',(0.707917883896095,-0.246942143572133,
0.679352081686668));
#15870=CARTESIAN_POINT('Ctrl Pts',(0.722929908501543,-0.244251601209411,
0.663382628119203));
#15871=CARTESIAN_POINT('Ctrl Pts',(0.750785745543687,-0.232861760990032,
0.631684198665439));
#15872=CARTESIAN_POINT('Ctrl Pts',(0.763642258217232,-0.224161999508995,
0.615966552324775));
#15873=CARTESIAN_POINT('Ctrl Pts',(0.78555112003688,-0.203463743702801,
0.587792702767295));
#15874=CARTESIAN_POINT('Ctrl Pts',(0.795684265985088,-0.190326085855194,
0.573915184558108));
#15875=CARTESIAN_POINT('Ctrl Pts',(0.813159949759,-0.15976606450048,0.548874290046456));
#15876=CARTESIAN_POINT('Ctrl Pts',(0.820511285096538,-0.142345102874864,
0.537715343527944));
#15877=CARTESIAN_POINT('Ctrl Pts',(0.833661031856294,-0.099930567888331,
0.517157748491653));
#15878=CARTESIAN_POINT('Ctrl Pts',(0.838633903678357,-0.0740444353928835,
0.508899795931835));
#15879=CARTESIAN_POINT('Ctrl Pts',(0.841298510752801,-0.0476299999999999,
0.504455939115715));
#15880=CARTESIAN_POINT('',(0.528110872004958,-0.04763,0.871530771444223));
#15881=CARTESIAN_POINT('Origin',(0.707106781186547,-0.04763,0.707106781186548));
#15882=CARTESIAN_POINT('',(0.871530771444223,-0.04763,0.528110872004959));
#15883=CARTESIAN_POINT('Ctrl Pts',(0.871530771444223,-0.0476300000000001,
0.528110872004958));
#15884=CARTESIAN_POINT('Ctrl Pts',(0.87014664509073,-0.0609922781173483,
0.530395067942936));
#15885=CARTESIAN_POINT('Ctrl Pts',(0.868149331745851,-0.0742967091364493,
0.533674141594226));
#15886=CARTESIAN_POINT('Ctrl Pts',(0.85981294420286,-0.115492077056649,
0.54708917182331));
#15887=CARTESIAN_POINT('Ctrl Pts',(0.850993704737257,-0.141695629206859,
0.560922177770136));
#15888=CARTESIAN_POINT('Ctrl Pts',(0.830754510485543,-0.181890537957859,
0.590422647829571));
#15889=CARTESIAN_POINT('Ctrl Pts',(0.816896541396381,-0.201072148666545,
0.609616703125488));
#15890=CARTESIAN_POINT('Ctrl Pts',(0.792310597819928,-0.223955109275652,
0.641117951819998));
#15891=CARTESIAN_POINT('Ctrl Pts',(0.779109323683612,-0.232742381310829,
0.657208095763053));
#15892=CARTESIAN_POINT('Ctrl Pts',(0.750552691816206,-0.244234834628584,
0.68964083160521));
#15893=CARTESIAN_POINT('Ctrl Pts',(0.735185187071673,-0.246942143572133,
0.705971972091755));
#15894=CARTESIAN_POINT('Ctrl Pts',(0.705971972091754,-0.246942143572133,
0.735185187071673));
#15895=CARTESIAN_POINT('Ctrl Pts',(0.689640831605209,-0.244234834628584,
0.750552691816206));
#15896=CARTESIAN_POINT('Ctrl Pts',(0.657208095763052,-0.232742381310829,
0.779109323683612));
#15897=CARTESIAN_POINT('Ctrl Pts',(0.641117951819998,-0.223955109275652,
0.792310597819928));
#15898=CARTESIAN_POINT('Ctrl Pts',(0.609616703125487,-0.201072148666545,
0.816896541396382));
#15899=CARTESIAN_POINT('Ctrl Pts',(0.590422647829571,-0.181890537957858,
0.830754510485544));
#15900=CARTESIAN_POINT('Ctrl Pts',(0.560922177770135,-0.141695629206858,
0.850993704737257));
#15901=CARTESIAN_POINT('Ctrl Pts',(0.547089171823309,-0.115492077056649,
0.859812944202861));
#15902=CARTESIAN_POINT('Ctrl Pts',(0.533674141594226,-0.0742967091364491,
0.868149331745852));
#15903=CARTESIAN_POINT('Ctrl Pts',(0.530395067942936,-0.0609922781173483,
0.870146645090731));
#15904=CARTESIAN_POINT('Ctrl Pts',(0.528110872004958,-0.0476300000000001,
0.871530771444223));
#15905=CARTESIAN_POINT('Origin',(0.707106781186547,-0.04763,0.707106781186548));
#15906=CARTESIAN_POINT('Origin',(0.,-0.166705,0.));
#15907=CARTESIAN_POINT('',(0.242834539687906,-0.04763,0.989696097314));
#15908=CARTESIAN_POINT('Origin',(0.,-0.04763,0.));
#15909=CARTESIAN_POINT('',(-0.242834539687907,-0.04763,0.989696097314));
#15910=CARTESIAN_POINT('Ctrl Pts',(0.242834539687906,-0.04763,0.989696097314));
#15911=CARTESIAN_POINT('Ctrl Pts',(0.24024064412003,-0.0609922781173483,
0.990332542620729));
#15912=CARTESIAN_POINT('Ctrl Pts',(0.236509675094874,-0.0742967091364492,
0.991238884025248));
#15913=CARTESIAN_POINT('Ctrl Pts',(0.221129100087819,-0.115492077056649,
0.994830026707808));
#15914=CARTESIAN_POINT('Ctrl Pts',(0.205111543747588,-0.141695629206859,
0.998375294985966));
#15915=CARTESIAN_POINT('Ctrl Pts',(0.169940289819232,-0.181890537957859,
1.00492400591205));
#15916=CARTESIAN_POINT('Ctrl Pts',(0.1465689792446,-0.201072148666545,1.00869718865384));
#15917=CARTESIAN_POINT('Ctrl Pts',(0.106909345252087,-0.223955109275652,
1.01358704779679));
#15918=CARTESIAN_POINT('Ctrl Pts',(0.0861971848975941,-0.232742381310829,
1.0156297872271));
#15919=CARTESIAN_POINT('Ctrl Pts',(0.0430711894098822,-0.244234834628584,
1.01837060663223));
#15920=CARTESIAN_POINT('Ctrl Pts',(0.0206568624125605,-0.246942143572133,
1.019052));
#15921=CARTESIAN_POINT('Ctrl Pts',(-0.0206568624125608,-0.246942143572133,
1.019052));
#15922=CARTESIAN_POINT('Ctrl Pts',(-0.0430711894098825,-0.244234834628584,
1.01837060663223));
#15923=CARTESIAN_POINT('Ctrl Pts',(-0.0861971848975943,-0.232742381310829,
1.0156297872271));
#15924=CARTESIAN_POINT('Ctrl Pts',(-0.106909345252088,-0.223955109275652,
1.01358704779679));
#15925=CARTESIAN_POINT('Ctrl Pts',(-0.1465689792446,-0.201072148666545,
1.00869718865384));
#15926=CARTESIAN_POINT('Ctrl Pts',(-0.169940289819232,-0.181890537957859,
1.00492400591205));
#15927=CARTESIAN_POINT('Ctrl Pts',(-0.205111543747588,-0.141695629206859,
0.998375294985966));
#15928=CARTESIAN_POINT('Ctrl Pts',(-0.221129100087819,-0.115492077056649,
0.994830026707808));
#15929=CARTESIAN_POINT('Ctrl Pts',(-0.236509675094875,-0.0742967091364493,
0.991238884025248));
#15930=CARTESIAN_POINT('Ctrl Pts',(-0.24024064412003,-0.0609922781173483,
0.990332542620729));
#15931=CARTESIAN_POINT('Ctrl Pts',(-0.242834539687907,-0.04763,0.989696097314));
#15932=CARTESIAN_POINT('',(-0.528110872004959,-0.04763,0.871530771444223));
#15933=CARTESIAN_POINT('Origin',(0.,-0.04763,0.));
#15934=CARTESIAN_POINT('',(-0.871530771444223,-0.04763,0.528110872004958));
#15935=CARTESIAN_POINT('Ctrl Pts',(-0.528110872004958,-0.0476300000000001,
0.871530771444223));
#15936=CARTESIAN_POINT('Ctrl Pts',(-0.530395067942936,-0.0609922781173484,
0.87014664509073));
#15937=CARTESIAN_POINT('Ctrl Pts',(-0.533674141594226,-0.0742967091364493,
0.868149331745851));
#15938=CARTESIAN_POINT('Ctrl Pts',(-0.54708917182331,-0.115492077056649,
0.85981294420286));
#15939=CARTESIAN_POINT('Ctrl Pts',(-0.560922177770136,-0.141695629206859,
0.850993704737257));
#15940=CARTESIAN_POINT('Ctrl Pts',(-0.590422647829571,-0.181890537957859,
0.830754510485543));
#15941=CARTESIAN_POINT('Ctrl Pts',(-0.609616703125488,-0.201072148666545,
0.816896541396381));
#15942=CARTESIAN_POINT('Ctrl Pts',(-0.641117951819998,-0.223955109275652,
0.792310597819928));
#15943=CARTESIAN_POINT('Ctrl Pts',(-0.657208095763053,-0.232742381310829,
0.779109323683611));
#15944=CARTESIAN_POINT('Ctrl Pts',(-0.68964083160521,-0.244234834628584,
0.750552691816205));
#15945=CARTESIAN_POINT('Ctrl Pts',(-0.705971972091755,-0.246942143572133,
0.735185187071673));
#15946=CARTESIAN_POINT('Ctrl Pts',(-0.735185187071673,-0.246942143572133,
0.705971972091754));
#15947=CARTESIAN_POINT('Ctrl Pts',(-0.750552691816206,-0.244234834628584,
0.689640831605209));
#15948=CARTESIAN_POINT('Ctrl Pts',(-0.779109323683612,-0.232742381310829,
0.657208095763052));
#15949=CARTESIAN_POINT('Ctrl Pts',(-0.792310597819928,-0.223955109275652,
0.641117951819998));
#15950=CARTESIAN_POINT('Ctrl Pts',(-0.816896541396382,-0.201072148666545,
0.609616703125487));
#15951=CARTESIAN_POINT('Ctrl Pts',(-0.830754510485544,-0.181890537957858,
0.590422647829571));
#15952=CARTESIAN_POINT('Ctrl Pts',(-0.850993704737257,-0.141695629206858,
0.560922177770135));
#15953=CARTESIAN_POINT('Ctrl Pts',(-0.859812944202861,-0.115492077056649,
0.547089171823309));
#15954=CARTESIAN_POINT('Ctrl Pts',(-0.868149331745852,-0.0742967091364491,
0.533674141594226));
#15955=CARTESIAN_POINT('Ctrl Pts',(-0.870146645090731,-0.0609922781173483,
0.530395067942936));
#15956=CARTESIAN_POINT('Ctrl Pts',(-0.871530771444223,-0.04763,0.528110872004958));
#15957=CARTESIAN_POINT('',(-0.989696097314,-0.04763,0.242834539687906));
#15958=CARTESIAN_POINT('Origin',(0.,-0.04763,0.));
#15959=CARTESIAN_POINT('',(-1.019052,-0.246942143572133,1.248489836334E-16));
#15960=CARTESIAN_POINT('Ctrl Pts',(-0.989696097314,-0.04763,0.242834539687906));
#15961=CARTESIAN_POINT('Ctrl Pts',(-0.990332542620729,-0.0609922781173483,
0.24024064412003));
#15962=CARTESIAN_POINT('Ctrl Pts',(-0.991238884025248,-0.0742967091364492,
0.236509675094874));
#15963=CARTESIAN_POINT('Ctrl Pts',(-0.994830026707808,-0.115492077056649,
0.221129100087819));
#15964=CARTESIAN_POINT('Ctrl Pts',(-0.998375294985966,-0.141695629206859,
0.205111543747588));
#15965=CARTESIAN_POINT('Ctrl Pts',(-1.00492400591205,-0.181890537957859,
0.169940289819232));
#15966=CARTESIAN_POINT('Ctrl Pts',(-1.00869718865384,-0.201072148666545,
0.1465689792446));
#15967=CARTESIAN_POINT('Ctrl Pts',(-1.01358704779679,-0.223955109275652,
0.106909345252088));
#15968=CARTESIAN_POINT('Ctrl Pts',(-1.0156297872271,-0.232742381310829,
0.0861971848975944));
#15969=CARTESIAN_POINT('Ctrl Pts',(-1.01837060663223,-0.244234834628584,
0.0430711894098825));
#15970=CARTESIAN_POINT('Ctrl Pts',(-1.019052,-0.246942143572133,0.0206568624125608));
#15971=CARTESIAN_POINT('Ctrl Pts',(-1.019052,-0.246942143572133,1.2490009027033E-16));
#15972=CARTESIAN_POINT('',(-1.019052,-0.28578,1.24797876996471E-16));
#15973=CARTESIAN_POINT('',(-1.019052,-0.166705,1.24797876996471E-16));
#15974=CARTESIAN_POINT('Origin',(0.,-0.28578,0.));
#15975=CARTESIAN_POINT('',(-0.989696097314,-0.04763,-0.242834539687906));
#15976=CARTESIAN_POINT('Ctrl Pts',(-1.019052,-0.246942143572133,1.2490009027033E-16));
#15977=CARTESIAN_POINT('Ctrl Pts',(-1.019052,-0.246942143572133,-0.0206568624125605));
#15978=CARTESIAN_POINT('Ctrl Pts',(-1.01837060663223,-0.244234834628584,
-0.0430711894098822));
#15979=CARTESIAN_POINT('Ctrl Pts',(-1.0156297872271,-0.232742381310829,
-0.0861971848975941));
#15980=CARTESIAN_POINT('Ctrl Pts',(-1.01358704779679,-0.223955109275652,
-0.106909345252087));
#15981=CARTESIAN_POINT('Ctrl Pts',(-1.00869718865384,-0.201072148666546,
-0.1465689792446));
#15982=CARTESIAN_POINT('Ctrl Pts',(-1.00492400591205,-0.181890537957859,
-0.169940289819232));
#15983=CARTESIAN_POINT('Ctrl Pts',(-0.998375294985966,-0.141695629206859,
-0.205111543747588));
#15984=CARTESIAN_POINT('Ctrl Pts',(-0.994830026707808,-0.11549207705665,
-0.221129100087819));
#15985=CARTESIAN_POINT('Ctrl Pts',(-0.991238884025248,-0.0742967091364495,
-0.236509675094874));
#15986=CARTESIAN_POINT('Ctrl Pts',(-0.990332542620729,-0.0609922781173484,
-0.24024064412003));
#15987=CARTESIAN_POINT('Ctrl Pts',(-0.989696097314,-0.0476300000000001,
-0.242834539687907));
#15988=CARTESIAN_POINT('',(-0.871530771444223,-0.04763,-0.528110872004958));
#15989=CARTESIAN_POINT('Origin',(0.,-0.04763,0.));
#15990=CARTESIAN_POINT('',(-0.528110872004958,-0.04763,-0.871530771444223));
#15991=CARTESIAN_POINT('Ctrl Pts',(-0.871530771444223,-0.0476300000000001,
-0.528110872004958));
#15992=CARTESIAN_POINT('Ctrl Pts',(-0.87014664509073,-0.0609922781173484,
-0.530395067942936));
#15993=CARTESIAN_POINT('Ctrl Pts',(-0.868149331745851,-0.0742967091364494,
-0.533674141594226));
#15994=CARTESIAN_POINT('Ctrl Pts',(-0.85981294420286,-0.115492077056649,
-0.54708917182331));
#15995=CARTESIAN_POINT('Ctrl Pts',(-0.850993704737257,-0.141695629206859,
-0.560922177770136));
#15996=CARTESIAN_POINT('Ctrl Pts',(-0.830754510485543,-0.181890537957859,
-0.590422647829571));
#15997=CARTESIAN_POINT('Ctrl Pts',(-0.816896541396381,-0.201072148666546,
-0.609616703125488));
#15998=CARTESIAN_POINT('Ctrl Pts',(-0.792310597819928,-0.223955109275652,
-0.641117951819999));
#15999=CARTESIAN_POINT('Ctrl Pts',(-0.779109323683611,-0.232742381310829,
-0.657208095763053));
#16000=CARTESIAN_POINT('Ctrl Pts',(-0.750552691816205,-0.244234834628584,
-0.68964083160521));
#16001=CARTESIAN_POINT('Ctrl Pts',(-0.735185187071673,-0.246942143572133,
-0.705971972091755));
#16002=CARTESIAN_POINT('Ctrl Pts',(-0.705971972091754,-0.246942143572133,
-0.735185187071673));
#16003=CARTESIAN_POINT('Ctrl Pts',(-0.68964083160521,-0.244234834628584,
-0.750552691816206));
#16004=CARTESIAN_POINT('Ctrl Pts',(-0.657208095763052,-0.232742381310829,
-0.779109323683612));
#16005=CARTESIAN_POINT('Ctrl Pts',(-0.641117951819998,-0.223955109275652,
-0.792310597819928));
#16006=CARTESIAN_POINT('Ctrl Pts',(-0.609616703125488,-0.201072148666545,
-0.816896541396381));
#16007=CARTESIAN_POINT('Ctrl Pts',(-0.590422647829571,-0.181890537957859,
-0.830754510485543));
#16008=CARTESIAN_POINT('Ctrl Pts',(-0.560922177770136,-0.141695629206859,
-0.850993704737257));
#16009=CARTESIAN_POINT('Ctrl Pts',(-0.54708917182331,-0.115492077056649,
-0.85981294420286));
#16010=CARTESIAN_POINT('Ctrl Pts',(-0.533674141594226,-0.0742967091364494,
-0.868149331745852));
#16011=CARTESIAN_POINT('Ctrl Pts',(-0.530395067942936,-0.0609922781173484,
-0.870146645090731));
#16012=CARTESIAN_POINT('Ctrl Pts',(-0.528110872004958,-0.0476300000000001,
-0.871530771444223));
#16013=CARTESIAN_POINT('',(-0.242834539687906,-0.04763,-0.989696097314));
#16014=CARTESIAN_POINT('Origin',(0.,-0.04763,0.));
#16015=CARTESIAN_POINT('',(0.242834539687906,-0.04763,-0.989696097314));
#16016=CARTESIAN_POINT('Ctrl Pts',(-0.242834539687907,-0.04763,-0.989696097314));
#16017=CARTESIAN_POINT('Ctrl Pts',(-0.24024064412003,-0.0609922781173483,
-0.990332542620729));
#16018=CARTESIAN_POINT('Ctrl Pts',(-0.236509675094874,-0.0742967091364493,
-0.991238884025248));
#16019=CARTESIAN_POINT('Ctrl Pts',(-0.221129100087819,-0.115492077056649,
-0.994830026707808));
#16020=CARTESIAN_POINT('Ctrl Pts',(-0.205111543747588,-0.141695629206859,
-0.998375294985966));
#16021=CARTESIAN_POINT('Ctrl Pts',(-0.169940289819232,-0.181890537957859,
-1.00492400591205));
#16022=CARTESIAN_POINT('Ctrl Pts',(-0.1465689792446,-0.201072148666545,
-1.00869718865384));
#16023=CARTESIAN_POINT('Ctrl Pts',(-0.106909345252087,-0.223955109275652,
-1.01358704779679));
#16024=CARTESIAN_POINT('Ctrl Pts',(-0.0861971848975942,-0.232742381310829,
-1.0156297872271));
#16025=CARTESIAN_POINT('Ctrl Pts',(-0.0430711894098823,-0.244234834628584,
-1.01837060663223));
#16026=CARTESIAN_POINT('Ctrl Pts',(-0.0206568624125606,-0.246942143572133,
-1.019052));
#16027=CARTESIAN_POINT('Ctrl Pts',(0.0206568624125607,-0.246942143572133,
-1.019052));
#16028=CARTESIAN_POINT('Ctrl Pts',(0.0430711894098824,-0.244234834628584,
-1.01837060663223));
#16029=CARTESIAN_POINT('Ctrl Pts',(0.0861971848975943,-0.232742381310829,
-1.0156297872271));
#16030=CARTESIAN_POINT('Ctrl Pts',(0.106909345252088,-0.223955109275652,
-1.01358704779679));
#16031=CARTESIAN_POINT('Ctrl Pts',(0.1465689792446,-0.201072148666545,-1.00869718865384));
#16032=CARTESIAN_POINT('Ctrl Pts',(0.169940289819232,-0.181890537957859,
-1.00492400591205));
#16033=CARTESIAN_POINT('Ctrl Pts',(0.205111543747588,-0.141695629206859,
-0.998375294985966));
#16034=CARTESIAN_POINT('Ctrl Pts',(0.221129100087819,-0.115492077056649,
-0.994830026707808));
#16035=CARTESIAN_POINT('Ctrl Pts',(0.236509675094874,-0.0742967091364493,
-0.991238884025248));
#16036=CARTESIAN_POINT('Ctrl Pts',(0.24024064412003,-0.0609922781173484,
-0.990332542620729));
#16037=CARTESIAN_POINT('Ctrl Pts',(0.242834539687907,-0.04763,-0.989696097314));
#16038=CARTESIAN_POINT('',(0.528110872004958,-0.04763,-0.871530771444223));
#16039=CARTESIAN_POINT('Origin',(0.,-0.04763,0.));
#16040=CARTESIAN_POINT('',(0.871530771444223,-0.04763,-0.528110872004958));
#16041=CARTESIAN_POINT('Ctrl Pts',(0.528110872004958,-0.0476300000000001,
-0.871530771444223));
#16042=CARTESIAN_POINT('Ctrl Pts',(0.530395067942936,-0.0609922781173484,
-0.870146645090731));
#16043=CARTESIAN_POINT('Ctrl Pts',(0.533674141594226,-0.0742967091364493,
-0.868149331745851));
#16044=CARTESIAN_POINT('Ctrl Pts',(0.54708917182331,-0.115492077056649,
-0.85981294420286));
#16045=CARTESIAN_POINT('Ctrl Pts',(0.560922177770136,-0.141695629206859,
-0.850993704737257));
#16046=CARTESIAN_POINT('Ctrl Pts',(0.590422647829571,-0.181890537957859,
-0.830754510485543));
#16047=CARTESIAN_POINT('Ctrl Pts',(0.609616703125488,-0.201072148666545,
-0.816896541396381));
#16048=CARTESIAN_POINT('Ctrl Pts',(0.641117951819998,-0.223955109275652,
-0.792310597819928));
#16049=CARTESIAN_POINT('Ctrl Pts',(0.657208095763053,-0.232742381310829,
-0.779109323683612));
#16050=CARTESIAN_POINT('Ctrl Pts',(0.68964083160521,-0.244234834628584,
-0.750552691816206));
#16051=CARTESIAN_POINT('Ctrl Pts',(0.705971972091755,-0.246942143572133,
-0.735185187071673));
#16052=CARTESIAN_POINT('Ctrl Pts',(0.735185187071673,-0.246942143572133,
-0.705971972091754));
#16053=CARTESIAN_POINT('Ctrl Pts',(0.750552691816206,-0.244234834628584,
-0.68964083160521));
#16054=CARTESIAN_POINT('Ctrl Pts',(0.779109323683612,-0.232742381310829,
-0.657208095763053));
#16055=CARTESIAN_POINT('Ctrl Pts',(0.792310597819928,-0.223955109275652,
-0.641117951819998));
#16056=CARTESIAN_POINT('Ctrl Pts',(0.816896541396381,-0.201072148666545,
-0.609616703125488));
#16057=CARTESIAN_POINT('Ctrl Pts',(0.830754510485543,-0.181890537957859,
-0.590422647829571));
#16058=CARTESIAN_POINT('Ctrl Pts',(0.850993704737257,-0.141695629206859,
-0.560922177770136));
#16059=CARTESIAN_POINT('Ctrl Pts',(0.85981294420286,-0.115492077056649,
-0.54708917182331));
#16060=CARTESIAN_POINT('Ctrl Pts',(0.868149331745851,-0.0742967091364493,
-0.533674141594226));
#16061=CARTESIAN_POINT('Ctrl Pts',(0.870146645090731,-0.0609922781173484,
-0.530395067942936));
#16062=CARTESIAN_POINT('Ctrl Pts',(0.871530771444223,-0.0476300000000001,
-0.528110872004958));
#16063=CARTESIAN_POINT('',(0.989696097314,-0.04763,-0.242834539687906));
#16064=CARTESIAN_POINT('Origin',(0.,-0.04763,0.));
#16065=CARTESIAN_POINT('',(0.989696097314,-0.04763,0.242834539687906));
#16066=CARTESIAN_POINT('Ctrl Pts',(0.989696097314,-0.04763,-0.242834539687907));
#16067=CARTESIAN_POINT('Ctrl Pts',(0.990332542620729,-0.0609922781173483,
-0.24024064412003));
#16068=CARTESIAN_POINT('Ctrl Pts',(0.991238884025248,-0.0742967091364493,
-0.236509675094874));
#16069=CARTESIAN_POINT('Ctrl Pts',(0.994830026707808,-0.115492077056649,
-0.221129100087819));
#16070=CARTESIAN_POINT('Ctrl Pts',(0.998375294985966,-0.141695629206859,
-0.205111543747588));
#16071=CARTESIAN_POINT('Ctrl Pts',(1.00492400591205,-0.181890537957859,
-0.169940289819232));
#16072=CARTESIAN_POINT('Ctrl Pts',(1.00869718865384,-0.201072148666545,
-0.1465689792446));
#16073=CARTESIAN_POINT('Ctrl Pts',(1.01358704779679,-0.223955109275652,
-0.106909345252087));
#16074=CARTESIAN_POINT('Ctrl Pts',(1.0156297872271,-0.232742381310829,-0.0861971848975942));
#16075=CARTESIAN_POINT('Ctrl Pts',(1.01837060663223,-0.244234834628584,
-0.0430711894098823));
#16076=CARTESIAN_POINT('Ctrl Pts',(1.019052,-0.246942143572133,-0.0206568624125607));
#16077=CARTESIAN_POINT('Ctrl Pts',(1.019052,-0.246942143572133,0.0206568624125607));
#16078=CARTESIAN_POINT('Ctrl Pts',(1.01837060663223,-0.244234834628584,
0.0430711894098823));
#16079=CARTESIAN_POINT('Ctrl Pts',(1.0156297872271,-0.232742381310829,0.0861971848975942));
#16080=CARTESIAN_POINT('Ctrl Pts',(1.01358704779679,-0.223955109275652,
0.106909345252087));
#16081=CARTESIAN_POINT('Ctrl Pts',(1.00869718865384,-0.201072148666545,
0.1465689792446));
#16082=CARTESIAN_POINT('Ctrl Pts',(1.00492400591205,-0.181890537957859,
0.169940289819232));
#16083=CARTESIAN_POINT('Ctrl Pts',(0.998375294985966,-0.141695629206859,
0.205111543747588));
#16084=CARTESIAN_POINT('Ctrl Pts',(0.994830026707808,-0.115492077056649,
0.221129100087819));
#16085=CARTESIAN_POINT('Ctrl Pts',(0.991238884025248,-0.0742967091364492,
0.236509675094874));
#16086=CARTESIAN_POINT('Ctrl Pts',(0.990332542620729,-0.0609922781173483,
0.24024064412003));
#16087=CARTESIAN_POINT('Ctrl Pts',(0.989696097314,-0.04763,0.242834539687907));
#16088=CARTESIAN_POINT('Origin',(0.,-0.04763,0.));
#16089=CARTESIAN_POINT('Origin',(0.,-0.04763,0.));
#16090=CARTESIAN_POINT('',(0.238183666596899,-0.04763,0.951592097314));
#16091=CARTESIAN_POINT('Origin',(0.,-0.04763,0.));
#16092=CARTESIAN_POINT('Origin',(-1.94289029309402E-16,-0.04763,1.));
#16093=CARTESIAN_POINT('Origin',(-1.94289029309402E-16,0.,1.));
#16094=CARTESIAN_POINT('',(-0.2381836665969,-0.04763,0.951592097314));
#16095=CARTESIAN_POINT('Ctrl Pts',(-0.238183666596899,-0.0476299999999999,
0.951592097314));
#16096=CARTESIAN_POINT('Ctrl Pts',(-0.233157223576062,-0.0740444353928835,
0.952850216871763));
#16097=CARTESIAN_POINT('Ctrl Pts',(-0.223801617934946,-0.0999305678883309,
0.955173119738174));
#16098=CARTESIAN_POINT('Ctrl Pts',(-0.199966927975188,-0.142345102874864,
0.960411259488514));
#16099=CARTESIAN_POINT('Ctrl Pts',(-0.1868781821531,-0.159766064500479,
0.963103647174702));
#16100=CARTESIAN_POINT('Ctrl Pts',(-0.15681442133453,-0.190326085855194,
0.968453058988463));
#16101=CARTESIAN_POINT('Ctrl Pts',(-0.139836317888043,-0.203463743702801,
0.971100730005489));
#16102=CARTESIAN_POINT('Ctrl Pts',(-0.104422493053067,-0.224161999508995,
0.975530745318961));
#16103=CARTESIAN_POINT('Ctrl Pts',(-0.0842175114474176,-0.232861760990032,
0.977553872336861));
#16104=CARTESIAN_POINT('Ctrl Pts',(-0.0421062857595701,-0.244251601209411,
0.980270995488453));
#16105=CARTESIAN_POINT('Ctrl Pts',(-0.0201990724523197,-0.246942143572133,
0.980948));
#16106=CARTESIAN_POINT('Ctrl Pts',(0.020199072452319,-0.246942143572133,
0.980948));
#16107=CARTESIAN_POINT('Ctrl Pts',(0.0421062857595694,-0.244251601209411,
0.980270995488454));
#16108=CARTESIAN_POINT('Ctrl Pts',(0.0842175114474169,-0.232861760990032,
0.977553872336861));
#16109=CARTESIAN_POINT('Ctrl Pts',(0.104422493053067,-0.224161999508995,
0.975530745318961));
#16110=CARTESIAN_POINT('Ctrl Pts',(0.139836317888042,-0.203463743702801,
0.971100730005489));
#16111=CARTESIAN_POINT('Ctrl Pts',(0.15681442133453,-0.190326085855194,
0.968453058988463));
#16112=CARTESIAN_POINT('Ctrl Pts',(0.1868781821531,-0.15976606450048,0.963103647174702));
#16113=CARTESIAN_POINT('Ctrl Pts',(0.199966927975188,-0.142345102874864,
0.960411259488514));
#16114=CARTESIAN_POINT('Ctrl Pts',(0.223801617934945,-0.0999305678883309,
0.955173119738174));
#16115=CARTESIAN_POINT('Ctrl Pts',(0.233157223576061,-0.0740444353928835,
0.952850216871763));
#16116=CARTESIAN_POINT('Ctrl Pts',(0.238183666596899,-0.0476299999999999,
0.951592097314));
#16117=CARTESIAN_POINT('Origin',(-1.94289029309402E-16,-0.04763,1.));
#16118=CARTESIAN_POINT('Origin',(0.,-0.04763,0.));
#16119=CARTESIAN_POINT('',(-0.504455939115715,-0.04763,0.841298510752802));
#16120=CARTESIAN_POINT('Origin',(0.,-0.04763,0.));
#16121=CARTESIAN_POINT('Origin',(-0.707106781186548,-0.04763,0.707106781186547));
#16122=CARTESIAN_POINT('Origin',(-0.707106781186548,0.,0.707106781186547));
#16123=CARTESIAN_POINT('',(-0.841298510752802,-0.04763,0.504455939115715));
#16124=CARTESIAN_POINT('Ctrl Pts',(-0.841298510752802,-0.04763,0.504455939115715));
#16125=CARTESIAN_POINT('Ctrl Pts',(-0.838633903678357,-0.0740444353928835,
0.508899795931835));
#16126=CARTESIAN_POINT('Ctrl Pts',(-0.833661031856294,-0.0999305678883309,
0.517157748491652));
#16127=CARTESIAN_POINT('Ctrl Pts',(-0.820511285096538,-0.142345102874864,
0.537715343527944));
#16128=CARTESIAN_POINT('Ctrl Pts',(-0.813159949759,-0.159766064500479,0.548874290046456));
#16129=CARTESIAN_POINT('Ctrl Pts',(-0.795684265985089,-0.190326085855194,
0.573915184558107));
#16130=CARTESIAN_POINT('Ctrl Pts',(-0.78555112003688,-0.203463743702801,
0.587792702767295));
#16131=CARTESIAN_POINT('Ctrl Pts',(-0.763642258217233,-0.224161999508995,
0.615966552324775));
#16132=CARTESIAN_POINT('Ctrl Pts',(-0.750785745543687,-0.232861760990032,
0.631684198665438));
#16133=CARTESIAN_POINT('Ctrl Pts',(-0.722929908501543,-0.244251601209411,
0.663382628119203));
#16134=CARTESIAN_POINT('Ctrl Pts',(-0.707917883896095,-0.246942143572133,
0.679352081686668));
#16135=CARTESIAN_POINT('Ctrl Pts',(-0.679352081686668,-0.246942143572133,
0.707917883896095));
#16136=CARTESIAN_POINT('Ctrl Pts',(-0.663382628119203,-0.244251601209411,
0.722929908501544));
#16137=CARTESIAN_POINT('Ctrl Pts',(-0.631684198665438,-0.232861760990031,
0.750785745543687));
#16138=CARTESIAN_POINT('Ctrl Pts',(-0.615966552324775,-0.224161999508995,
0.763642258217233));
#16139=CARTESIAN_POINT('Ctrl Pts',(-0.587792702767295,-0.203463743702801,
0.78555112003688));
#16140=CARTESIAN_POINT('Ctrl Pts',(-0.573915184558107,-0.190326085855194,
0.795684265985088));
#16141=CARTESIAN_POINT('Ctrl Pts',(-0.548874290046456,-0.159766064500479,
0.813159949759));
#16142=CARTESIAN_POINT('Ctrl Pts',(-0.537715343527944,-0.142345102874864,
0.820511285096538));
#16143=CARTESIAN_POINT('Ctrl Pts',(-0.517157748491652,-0.0999305678883309,
0.833661031856294));
#16144=CARTESIAN_POINT('Ctrl Pts',(-0.508899795931835,-0.0740444353928835,
0.838633903678357));
#16145=CARTESIAN_POINT('Ctrl Pts',(-0.504455939115716,-0.04763,0.841298510752801));
#16146=CARTESIAN_POINT('Origin',(-0.707106781186548,-0.04763,0.707106781186547));
#16147=CARTESIAN_POINT('Origin',(0.,-0.04763,0.));
#16148=CARTESIAN_POINT('',(-0.951592097314,-0.04763,0.238183666596899));
#16149=CARTESIAN_POINT('Origin',(0.,-0.04763,0.));
#16150=CARTESIAN_POINT('Origin',(-1.,-0.04763,-1.11022302462516E-16));
#16151=CARTESIAN_POINT('Origin',(-1.,0.,-1.11022302462516E-16));
#16152=CARTESIAN_POINT('',(-0.951592097314,-0.04763,-0.2381836665969));
#16153=CARTESIAN_POINT('',(-0.980948,-0.246942143572133,1.08514323328844E-18));
#16154=CARTESIAN_POINT('Ctrl Pts',(-0.951592097314,-0.04763,-0.238183666596899));
#16155=CARTESIAN_POINT('Ctrl Pts',(-0.952850216871763,-0.0740444353928835,
-0.233157223576062));
#16156=CARTESIAN_POINT('Ctrl Pts',(-0.955173119738174,-0.0999305678883309,
-0.223801617934946));
#16157=CARTESIAN_POINT('Ctrl Pts',(-0.960411259488514,-0.142345102874864,
-0.199966927975188));
#16158=CARTESIAN_POINT('Ctrl Pts',(-0.963103647174702,-0.159766064500479,
-0.1868781821531));
#16159=CARTESIAN_POINT('Ctrl Pts',(-0.968453058988463,-0.190326085855194,
-0.15681442133453));
#16160=CARTESIAN_POINT('Ctrl Pts',(-0.971100730005489,-0.203463743702801,
-0.139836317888043));
#16161=CARTESIAN_POINT('Ctrl Pts',(-0.975530745318961,-0.224161999508995,
-0.104422493053067));
#16162=CARTESIAN_POINT('Ctrl Pts',(-0.977553872336861,-0.232861760990032,
-0.0842175114474175));
#16163=CARTESIAN_POINT('Ctrl Pts',(-0.980270995488453,-0.244251601209411,
-0.0421062857595699));
#16164=CARTESIAN_POINT('Ctrl Pts',(-0.980948,-0.246942143572133,-0.0201990724523195));
#16165=CARTESIAN_POINT('Ctrl Pts',(-0.980948,-0.246942143572133,-1.17961196366423E-16));
#16166=CARTESIAN_POINT('Origin',(-1.,-0.04763,-1.11022302462516E-16));
#16167=CARTESIAN_POINT('Ctrl Pts',(-0.980948,-0.246942143572133,-1.17961196366423E-16));
#16168=CARTESIAN_POINT('Ctrl Pts',(-0.980948,-0.246942143572133,0.0201990724523192));
#16169=CARTESIAN_POINT('Ctrl Pts',(-0.980270995488453,-0.244251601209411,
0.0421062857595695));
#16170=CARTESIAN_POINT('Ctrl Pts',(-0.977553872336861,-0.232861760990032,
0.0842175114474169));
#16171=CARTESIAN_POINT('Ctrl Pts',(-0.975530745318961,-0.224161999508995,
0.104422493053066));
#16172=CARTESIAN_POINT('Ctrl Pts',(-0.971100730005489,-0.203463743702801,
0.139836317888042));
#16173=CARTESIAN_POINT('Ctrl Pts',(-0.968453058988463,-0.190326085855194,
0.15681442133453));
#16174=CARTESIAN_POINT('Ctrl Pts',(-0.963103647174702,-0.15976606450048,
0.1868781821531));
#16175=CARTESIAN_POINT('Ctrl Pts',(-0.960411259488514,-0.142345102874864,
0.199966927975188));
#16176=CARTESIAN_POINT('Ctrl Pts',(-0.955173119738174,-0.099930567888331,
0.223801617934945));
#16177=CARTESIAN_POINT('Ctrl Pts',(-0.952850216871763,-0.0740444353928835,
0.233157223576061));
#16178=CARTESIAN_POINT('Ctrl Pts',(-0.951592097314,-0.04763,0.238183666596899));
#16179=CARTESIAN_POINT('Origin',(0.,-0.04763,0.));
#16180=CARTESIAN_POINT('',(-0.841298510752802,-0.04763,-0.504455939115715));
#16181=CARTESIAN_POINT('Origin',(0.,-0.04763,0.));
#16182=CARTESIAN_POINT('Origin',(-0.707106781186547,-0.04763,-0.707106781186548));
#16183=CARTESIAN_POINT('Origin',(-0.707106781186547,0.,-0.707106781186548));
#16184=CARTESIAN_POINT('',(-0.504455939115715,-0.04763,-0.841298510752802));
#16185=CARTESIAN_POINT('Ctrl Pts',(-0.504455939115715,-0.04763,-0.841298510752802));
#16186=CARTESIAN_POINT('Ctrl Pts',(-0.508899795931835,-0.0740444353928835,
-0.838633903678357));
#16187=CARTESIAN_POINT('Ctrl Pts',(-0.517157748491652,-0.0999305678883309,
-0.833661031856294));
#16188=CARTESIAN_POINT('Ctrl Pts',(-0.537715343527944,-0.142345102874864,
-0.820511285096538));
#16189=CARTESIAN_POINT('Ctrl Pts',(-0.548874290046456,-0.159766064500479,
-0.813159949759));
#16190=CARTESIAN_POINT('Ctrl Pts',(-0.573915184558107,-0.190326085855194,
-0.795684265985089));
#16191=CARTESIAN_POINT('Ctrl Pts',(-0.587792702767295,-0.203463743702801,
-0.78555112003688));
#16192=CARTESIAN_POINT('Ctrl Pts',(-0.615966552324775,-0.224161999508995,
-0.763642258217233));
#16193=CARTESIAN_POINT('Ctrl Pts',(-0.631684198665438,-0.232861760990032,
-0.750785745543687));
#16194=CARTESIAN_POINT('Ctrl Pts',(-0.663382628119203,-0.244251601209411,
-0.722929908501543));
#16195=CARTESIAN_POINT('Ctrl Pts',(-0.679352081686668,-0.246942143572133,
-0.707917883896095));
#16196=CARTESIAN_POINT('Ctrl Pts',(-0.707917883896095,-0.246942143572133,
-0.679352081686668));
#16197=CARTESIAN_POINT('Ctrl Pts',(-0.722929908501543,-0.244251601209411,
-0.663382628119203));
#16198=CARTESIAN_POINT('Ctrl Pts',(-0.750785745543687,-0.232861760990032,
-0.631684198665439));
#16199=CARTESIAN_POINT('Ctrl Pts',(-0.763642258217232,-0.224161999508995,
-0.615966552324775));
#16200=CARTESIAN_POINT('Ctrl Pts',(-0.78555112003688,-0.203463743702801,
-0.587792702767295));
#16201=CARTESIAN_POINT('Ctrl Pts',(-0.795684265985088,-0.190326085855194,
-0.573915184558107));
#16202=CARTESIAN_POINT('Ctrl Pts',(-0.813159949759,-0.15976606450048,-0.548874290046456));
#16203=CARTESIAN_POINT('Ctrl Pts',(-0.820511285096538,-0.142345102874864,
-0.537715343527944));
#16204=CARTESIAN_POINT('Ctrl Pts',(-0.833661031856294,-0.0999305678883311,
-0.517157748491652));
#16205=CARTESIAN_POINT('Ctrl Pts',(-0.838633903678357,-0.0740444353928836,
-0.508899795931835));
#16206=CARTESIAN_POINT('Ctrl Pts',(-0.841298510752801,-0.04763,-0.504455939115715));
#16207=CARTESIAN_POINT('Origin',(-0.707106781186547,-0.04763,-0.707106781186548));
#16208=CARTESIAN_POINT('Origin',(0.,-0.04763,0.));
#16209=CARTESIAN_POINT('',(-0.238183666596899,-0.04763,-0.951592097314));
#16210=CARTESIAN_POINT('Origin',(0.,-0.04763,0.));
#16211=CARTESIAN_POINT('Origin',(5.55111512312578E-17,-0.04763,-1.));
#16212=CARTESIAN_POINT('Origin',(5.55111512312578E-17,0.,-1.));
#16213=CARTESIAN_POINT('',(0.238183666596899,-0.04763,-0.951592097314));
#16214=CARTESIAN_POINT('Ctrl Pts',(0.238183666596899,-0.04763,-0.951592097314));
#16215=CARTESIAN_POINT('Ctrl Pts',(0.233157223576062,-0.0740444353928835,
-0.952850216871763));
#16216=CARTESIAN_POINT('Ctrl Pts',(0.223801617934946,-0.099930567888331,
-0.955173119738174));
#16217=CARTESIAN_POINT('Ctrl Pts',(0.199966927975188,-0.142345102874864,
-0.960411259488514));
#16218=CARTESIAN_POINT('Ctrl Pts',(0.1868781821531,-0.15976606450048,-0.963103647174702));
#16219=CARTESIAN_POINT('Ctrl Pts',(0.15681442133453,-0.190326085855194,
-0.968453058988463));
#16220=CARTESIAN_POINT('Ctrl Pts',(0.139836317888042,-0.203463743702801,
-0.971100730005489));
#16221=CARTESIAN_POINT('Ctrl Pts',(0.104422493053067,-0.224161999508995,
-0.975530745318961));
#16222=CARTESIAN_POINT('Ctrl Pts',(0.0842175114474173,-0.232861760990032,
-0.977553872336861));
#16223=CARTESIAN_POINT('Ctrl Pts',(0.0421062857595698,-0.244251601209411,
-0.980270995488453));
#16224=CARTESIAN_POINT('Ctrl Pts',(0.0201990724523194,-0.246942143572133,
-0.980948));
#16225=CARTESIAN_POINT('Ctrl Pts',(-0.0201990724523193,-0.246942143572133,
-0.980948));
#16226=CARTESIAN_POINT('Ctrl Pts',(-0.0421062857595697,-0.244251601209411,
-0.980270995488453));
#16227=CARTESIAN_POINT('Ctrl Pts',(-0.0842175114474171,-0.232861760990032,
-0.977553872336861));
#16228=CARTESIAN_POINT('Ctrl Pts',(-0.104422493053067,-0.224161999508995,
-0.975530745318961));
#16229=CARTESIAN_POINT('Ctrl Pts',(-0.139836317888042,-0.203463743702801,
-0.971100730005489));
#16230=CARTESIAN_POINT('Ctrl Pts',(-0.15681442133453,-0.190326085855194,
-0.968453058988463));
#16231=CARTESIAN_POINT('Ctrl Pts',(-0.1868781821531,-0.15976606450048,-0.963103647174702));
#16232=CARTESIAN_POINT('Ctrl Pts',(-0.199966927975188,-0.142345102874864,
-0.960411259488514));
#16233=CARTESIAN_POINT('Ctrl Pts',(-0.223801617934945,-0.099930567888331,
-0.955173119738174));
#16234=CARTESIAN_POINT('Ctrl Pts',(-0.233157223576062,-0.0740444353928835,
-0.952850216871763));
#16235=CARTESIAN_POINT('Ctrl Pts',(-0.238183666596899,-0.0476299999999999,
-0.951592097314));
#16236=CARTESIAN_POINT('Origin',(5.55111512312578E-17,-0.04763,-1.));
#16237=CARTESIAN_POINT('Origin',(0.,-0.04763,0.));
#16238=CARTESIAN_POINT('',(0.504455939115715,-0.04763,-0.841298510752802));
#16239=CARTESIAN_POINT('Origin',(0.,-0.04763,0.));
#16240=CARTESIAN_POINT('Origin',(0.707106781186548,-0.04763,-0.707106781186547));
#16241=CARTESIAN_POINT('Origin',(0.707106781186548,0.,-0.707106781186547));
#16242=CARTESIAN_POINT('',(0.841298510752802,-0.04763,-0.504455939115715));
#16243=CARTESIAN_POINT('Ctrl Pts',(0.841298510752802,-0.04763,-0.504455939115715));
#16244=CARTESIAN_POINT('Ctrl Pts',(0.838633903678357,-0.0740444353928835,
-0.508899795931835));
#16245=CARTESIAN_POINT('Ctrl Pts',(0.833661031856294,-0.0999305678883309,
-0.517157748491652));
#16246=CARTESIAN_POINT('Ctrl Pts',(0.820511285096538,-0.142345102874864,
-0.537715343527944));
#16247=CARTESIAN_POINT('Ctrl Pts',(0.813159949759,-0.159766064500479,-0.548874290046456));
#16248=CARTESIAN_POINT('Ctrl Pts',(0.795684265985088,-0.190326085855194,
-0.573915184558107));
#16249=CARTESIAN_POINT('Ctrl Pts',(0.78555112003688,-0.203463743702801,
-0.587792702767295));
#16250=CARTESIAN_POINT('Ctrl Pts',(0.763642258217233,-0.224161999508995,
-0.615966552324775));
#16251=CARTESIAN_POINT('Ctrl Pts',(0.750785745543687,-0.232861760990032,
-0.631684198665438));
#16252=CARTESIAN_POINT('Ctrl Pts',(0.722929908501543,-0.244251601209411,
-0.663382628119203));
#16253=CARTESIAN_POINT('Ctrl Pts',(0.707917883896095,-0.246942143572133,
-0.679352081686668));
#16254=CARTESIAN_POINT('Ctrl Pts',(0.679352081686668,-0.246942143572133,
-0.707917883896095));
#16255=CARTESIAN_POINT('Ctrl Pts',(0.663382628119203,-0.244251601209411,
-0.722929908501543));
#16256=CARTESIAN_POINT('Ctrl Pts',(0.631684198665438,-0.232861760990032,
-0.750785745543687));
#16257=CARTESIAN_POINT('Ctrl Pts',(0.615966552324775,-0.224161999508995,
-0.763642258217232));
#16258=CARTESIAN_POINT('Ctrl Pts',(0.587792702767295,-0.203463743702801,
-0.78555112003688));
#16259=CARTESIAN_POINT('Ctrl Pts',(0.573915184558107,-0.190326085855194,
-0.795684265985088));
#16260=CARTESIAN_POINT('Ctrl Pts',(0.548874290046456,-0.159766064500479,
-0.813159949759));
#16261=CARTESIAN_POINT('Ctrl Pts',(0.537715343527944,-0.142345102874864,
-0.820511285096538));
#16262=CARTESIAN_POINT('Ctrl Pts',(0.517157748491652,-0.099930567888331,
-0.833661031856294));
#16263=CARTESIAN_POINT('Ctrl Pts',(0.508899795931835,-0.0740444353928835,
-0.838633903678357));
#16264=CARTESIAN_POINT('Ctrl Pts',(0.504455939115715,-0.04763,-0.841298510752801));
#16265=CARTESIAN_POINT('Origin',(0.707106781186548,-0.04763,-0.707106781186547));
#16266=CARTESIAN_POINT('Origin',(0.,-0.166705,0.));
#16267=CARTESIAN_POINT('',(-0.980948,-0.28578,1.20131482833E-16));
#16268=CARTESIAN_POINT('Origin',(0.,-0.28578,0.));
#16269=CARTESIAN_POINT('',(-0.980948,-0.166705,1.20131482833E-16));
#16270=CARTESIAN_POINT('',(0.951592097314,-0.04763,0.238183666596899));
#16271=CARTESIAN_POINT('Origin',(0.,-0.04763,0.));
#16272=CARTESIAN_POINT('',(0.951592097314,-0.04763,-0.238183666596899));
#16273=CARTESIAN_POINT('Ctrl Pts',(0.951592097314,-0.04763,0.238183666596899));
#16274=CARTESIAN_POINT('Ctrl Pts',(0.952850216871763,-0.0740444353928835,
0.233157223576062));
#16275=CARTESIAN_POINT('Ctrl Pts',(0.955173119738174,-0.099930567888331,
0.223801617934945));
#16276=CARTESIAN_POINT('Ctrl Pts',(0.960411259488514,-0.142345102874864,
0.199966927975188));
#16277=CARTESIAN_POINT('Ctrl Pts',(0.963103647174702,-0.15976606450048,
0.1868781821531));
#16278=CARTESIAN_POINT('Ctrl Pts',(0.968453058988463,-0.190326085855194,
0.15681442133453));
#16279=CARTESIAN_POINT('Ctrl Pts',(0.971100730005489,-0.203463743702801,
0.139836317888042));
#16280=CARTESIAN_POINT('Ctrl Pts',(0.975530745318961,-0.224161999508995,
0.104422493053067));
#16281=CARTESIAN_POINT('Ctrl Pts',(0.977553872336861,-0.232861760990032,
0.0842175114474172));
#16282=CARTESIAN_POINT('Ctrl Pts',(0.980270995488453,-0.244251601209411,
0.0421062857595697));
#16283=CARTESIAN_POINT('Ctrl Pts',(0.980948,-0.246942143572133,0.0201990724523194));
#16284=CARTESIAN_POINT('Ctrl Pts',(0.980948,-0.246942143572133,-0.0201990724523194));
#16285=CARTESIAN_POINT('Ctrl Pts',(0.980270995488453,-0.244251601209411,
-0.0421062857595697));
#16286=CARTESIAN_POINT('Ctrl Pts',(0.977553872336861,-0.232861760990032,
-0.0842175114474172));
#16287=CARTESIAN_POINT('Ctrl Pts',(0.975530745318961,-0.224161999508995,
-0.104422493053067));
#16288=CARTESIAN_POINT('Ctrl Pts',(0.971100730005489,-0.203463743702801,
-0.139836317888042));
#16289=CARTESIAN_POINT('Ctrl Pts',(0.968453058988463,-0.190326085855194,
-0.15681442133453));
#16290=CARTESIAN_POINT('Ctrl Pts',(0.963103647174702,-0.15976606450048,
-0.1868781821531));
#16291=CARTESIAN_POINT('Ctrl Pts',(0.960411259488514,-0.142345102874864,
-0.199966927975188));
#16292=CARTESIAN_POINT('Ctrl Pts',(0.955173119738174,-0.099930567888331,
-0.223801617934945));
#16293=CARTESIAN_POINT('Ctrl Pts',(0.952850216871763,-0.0740444353928835,
-0.233157223576062));
#16294=CARTESIAN_POINT('Ctrl Pts',(0.951592097314,-0.0476299999999999,-0.238183666596899));
#16295=CARTESIAN_POINT('Origin',(0.,-0.04763,0.));
#16296=CARTESIAN_POINT('Origin',(0.,-0.04763,0.));
#16297=CARTESIAN_POINT('Origin',(1.,-0.04763,0.));
#16298=CARTESIAN_POINT('Origin',(1.,0.,0.));
#16299=CARTESIAN_POINT('Origin',(1.,-0.04763,0.));
#16300=CARTESIAN_POINT('Origin',(0.,-0.28578,0.));
#16301=CARTESIAN_POINT('Origin',(0.,-0.04763,0.));
#18931=UNCERTAINTY_MEASURE_WITH_UNIT(LENGTH_MEASURE(0.001),#19044,
'DISTANCE_ACCURACY_VALUE',
'Maximum model space distance between geometric entities at asserted c
onnectivities');
#18972=UNCERTAINTY_MEASURE_WITH_UNIT(LENGTH_MEASURE(0.001),#19044,
'DISTANCE_ACCURACY_VALUE',
'Maximum model space distance between geometric entities at asserted c
onnectivities');
#19002=(
GEOMETRIC_REPRESENTATION_CONTEXT(3)
GLOBAL_UNCERTAINTY_ASSIGNED_CONTEXT((#18931))
GLOBAL_UNIT_ASSIGNED_CONTEXT((#19044,#19046,#19047))
REPRESENTATION_CONTEXT('','3D')
);
#19043=(
GEOMETRIC_REPRESENTATION_CONTEXT(3)
GLOBAL_UNCERTAINTY_ASSIGNED_CONTEXT((#18972))
GLOBAL_UNIT_ASSIGNED_CONTEXT((#19044,#19046,#19047))
REPRESENTATION_CONTEXT('','3D')
);
#19044=(
LENGTH_UNIT()
NAMED_UNIT(*)
SI_UNIT(.CENTI.,.METRE.)
);
#19046=(
NAMED_UNIT(*)
PLANE_ANGLE_UNIT()
SI_UNIT($,.RADIAN.)
);
#19047=(
NAMED_UNIT(*)
SI_UNIT($,.STERADIAN.)
SOLID_ANGLE_UNIT()
);
#19077=SHAPE_DEFINITION_REPRESENTATION(#19147,#19335);
#19147=PRODUCT_DEFINITION_SHAPE('',$,#19406);
#19335=SHAPE_REPRESENTATION('',(#10762),#19002);
#19376=PRODUCT_DEFINITION_CONTEXT('part definition',#19588,'design');
#19406=PRODUCT_DEFINITION('2026-11-03-00-38-46-503','Cage',#19476,#19376);
#19476=PRODUCT_DEFINITION_FORMATION('',$,#19619);
#19588=APPLICATION_CONTEXT(
'Core Data for Automotive Mechanical Design Process');
#19589=PRODUCT_CONTEXT('part definition',#19588,'mechanical');
#19619=PRODUCT('2026-11-03-00-38-46-503','Cage','Cage',(#19589));
#19661=PRESENTATION_STYLE_ASSIGNMENT((#19667));
#19667=SURFACE_STYLE_USAGE(.BOTH.,#19673);
#19673=SURFACE_SIDE_STYLE('',(#19679));
#19679=SURFACE_STYLE_FILL_AREA(#19685);
#19685=FILL_AREA_STYLE('CAD Library Painted - Engineering blue',(#19691));
#19691=FILL_AREA_STYLE_COLOUR('CAD Library Painted - Engineering blue',
#19697);
#19697=COLOUR_RGB('CAD Library Painted - Engineering blue',0.12156862745098,
0.356862745098039,0.6);
ENDSEC;
END-ISO-10303-21;
